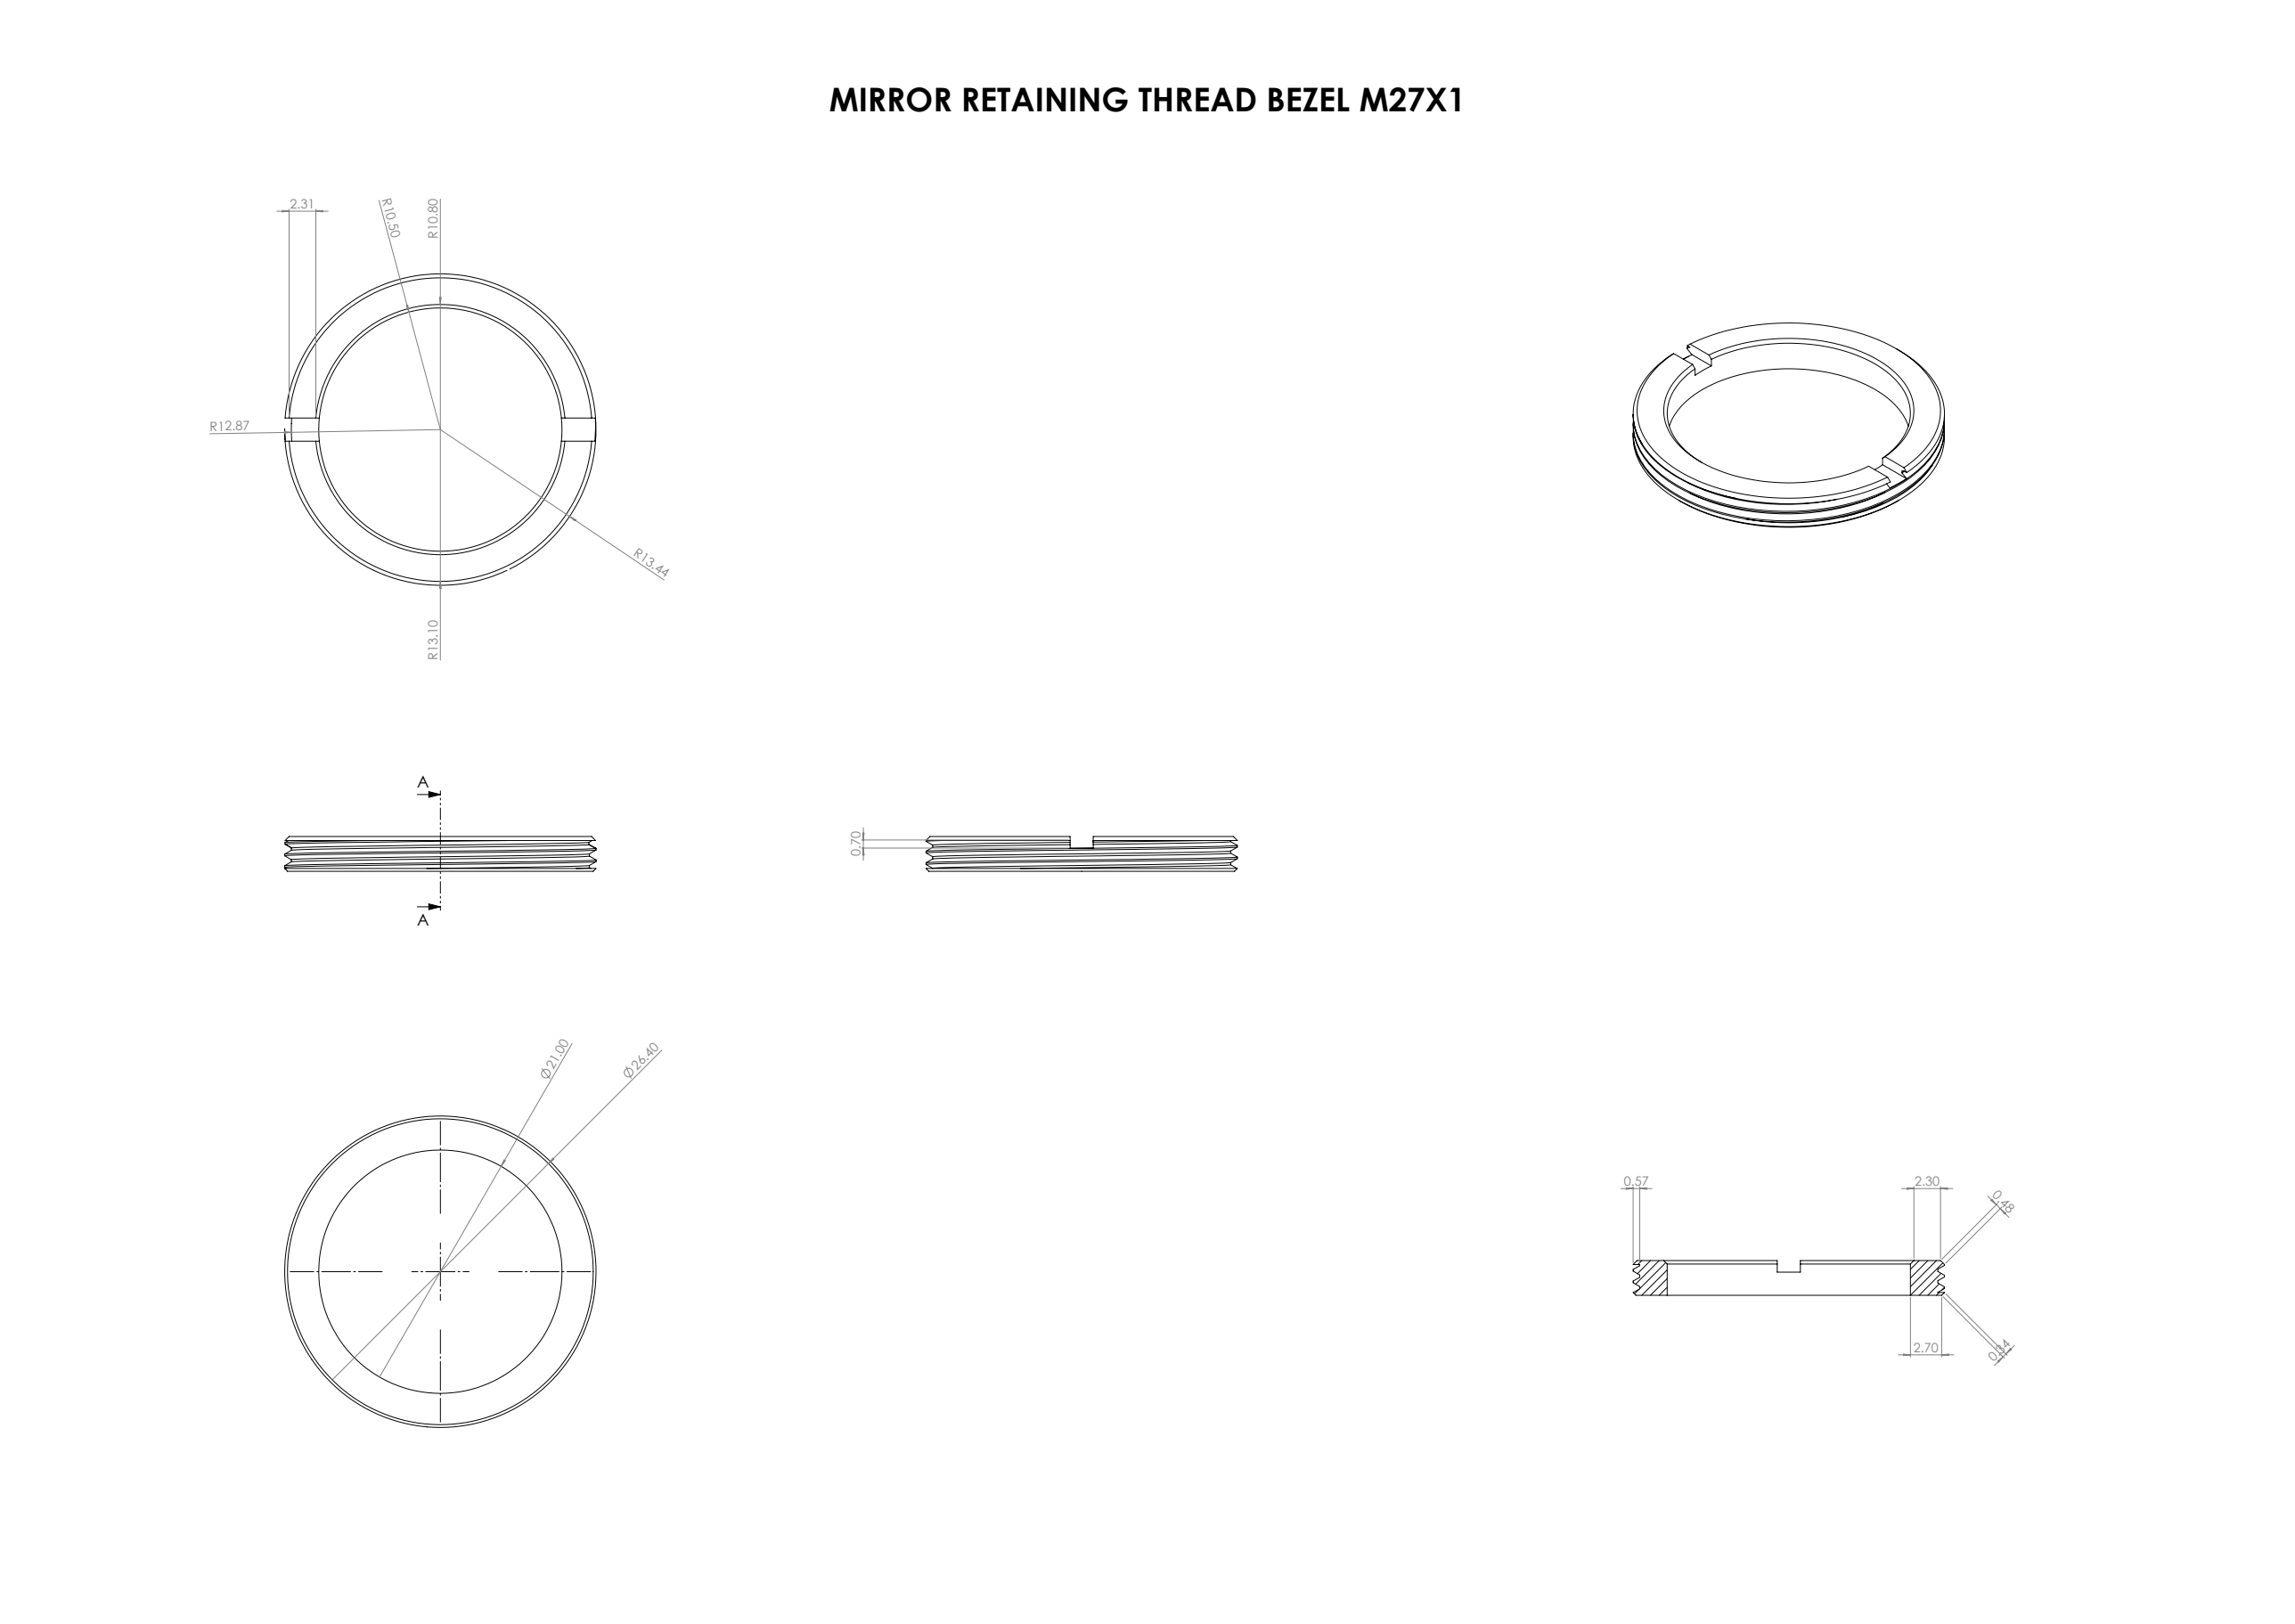
ISO-10303-21;
HEADER;
/* Generated by software containing ST-Developer
 * from STEP Tools, Inc. (www.steptools.com) 
 */

FILE_DESCRIPTION(
/* description */ (''),
/* implementation_level */ '2;1');

FILE_NAME(
/* name */ 
'07_Mirror_Retaining_Thread_Bezel_M27x1.step',
/* time_stamp */ '2026-10-20T10:06:23-07:00',
/* author */ (''),
/* organization */ (''),
/* preprocessor_version */ 'ST-DEVELOPER v20.2',
/* originating_system */ 'Autodesk Translation Framework v15.15.0.0',
/* authorisation */ '');

FILE_SCHEMA (('AUTOMOTIVE_DESIGN { 1 0 10303 214 3 1 1 }'));
ENDSEC;

DATA;
#10=MECHANICAL_DESIGN_GEOMETRIC_PRESENTATION_REPRESENTATION('',(#465),#38611);
#98=(
BOUNDED_CURVE()
B_SPLINE_CURVE(2,(#24495,#24496,#24497),.UNSPECIFIED.,.F.,.F.)
B_SPLINE_CURVE_WITH_KNOTS((3,3),(0.,0.048540461555457),.UNSPECIFIED.)
CURVE()
GEOMETRIC_REPRESENTATION_ITEM()
RATIONAL_B_SPLINE_CURVE((1.,1.0000974490119,1.00002789674321))
REPRESENTATION_ITEM('')
);
#99=(
BOUNDED_CURVE()
B_SPLINE_CURVE(2,(#24501,#24502,#24503),.UNSPECIFIED.,.F.,.F.)
B_SPLINE_CURVE_WITH_KNOTS((3,3),(0.,0.0425206671334367),.UNSPECIFIED.)
CURVE()
GEOMETRIC_REPRESENTATION_ITEM()
RATIONAL_B_SPLINE_CURVE((1.,1.00010008479633,1.))
REPRESENTATION_ITEM('')
);
#100=(
BOUNDED_CURVE()
B_SPLINE_CURVE(2,(#24513,#24514,#24515),.UNSPECIFIED.,.F.,.F.)
B_SPLINE_CURVE_WITH_KNOTS((3,3),(0.,0.0425206671334366),.UNSPECIFIED.)
CURVE()
GEOMETRIC_REPRESENTATION_ITEM()
RATIONAL_B_SPLINE_CURVE((1.,1.00010008445539,1.))
REPRESENTATION_ITEM('')
);
#101=(
BOUNDED_CURVE()
B_SPLINE_CURVE(2,(#24518,#24519,#24520),.UNSPECIFIED.,.F.,.F.)
B_SPLINE_CURVE_WITH_KNOTS((3,3),(0.00810844555795414,0.0566489071109945),
 .UNSPECIFIED.)
CURVE()
GEOMETRIC_REPRESENTATION_ITEM()
RATIONAL_B_SPLINE_CURVE((1.00002789660287,1.00009744852162,1.))
REPRESENTATION_ITEM('')
);
#102=(
BOUNDED_CURVE()
B_SPLINE_CURVE(2,(#24534,#24535,#24536),.UNSPECIFIED.,.F.,.F.)
B_SPLINE_CURVE_WITH_KNOTS((3,3),(0.,0.0485404615530411),.UNSPECIFIED.)
CURVE()
GEOMETRIC_REPRESENTATION_ITEM()
RATIONAL_B_SPLINE_CURVE((1.,1.00009744852162,1.00002789660287))
REPRESENTATION_ITEM('')
);
#103=(
BOUNDED_CURVE()
B_SPLINE_CURVE(2,(#24540,#24541,#24542),.UNSPECIFIED.,.F.,.F.)
B_SPLINE_CURVE_WITH_KNOTS((3,3),(0.,0.0425206671334366),.UNSPECIFIED.)
CURVE()
GEOMETRIC_REPRESENTATION_ITEM()
RATIONAL_B_SPLINE_CURVE((1.,1.00010008445539,1.))
REPRESENTATION_ITEM('')
);
#104=(
BOUNDED_CURVE()
B_SPLINE_CURVE(2,(#24552,#24553,#24554),.UNSPECIFIED.,.F.,.F.)
B_SPLINE_CURVE_WITH_KNOTS((3,3),(0.,0.0425206671334367),.UNSPECIFIED.)
CURVE()
GEOMETRIC_REPRESENTATION_ITEM()
RATIONAL_B_SPLINE_CURVE((1.,1.00010008479633,1.))
REPRESENTATION_ITEM('')
);
#105=(
BOUNDED_CURVE()
B_SPLINE_CURVE(2,(#24557,#24558,#24559),.UNSPECIFIED.,.F.,.F.)
B_SPLINE_CURVE_WITH_KNOTS((3,3),(0.00810844555553747,0.0566489071109946),
 .UNSPECIFIED.)
CURVE()
GEOMETRIC_REPRESENTATION_ITEM()
RATIONAL_B_SPLINE_CURVE((1.00002789674321,1.0000974490119,1.))
REPRESENTATION_ITEM('')
);
#437=SHAPE_REPRESENTATION_RELATIONSHIP('SRR','None',#38673,#451);
#451=ADVANCED_BREP_SHAPE_REPRESENTATION('',(#479),#38602);
#465=STYLED_ITEM('',(#38871),#479);
#479=MANIFOLD_SOLID_BREP('Ring',#16239);
#492=B_SPLINE_SURFACE_WITH_KNOTS('',3,3,((#23661,#23662,#23663,#23664,#23665,
#23666,#23667,#23668,#23669,#23670,#23671,#23672,#23673,#23674,#23675,#23676,
#23677,#23678,#23679,#23680,#23681,#23682,#23683,#23684,#23685,#23686,#23687,
#23688,#23689,#23690,#23691,#23692,#23693,#23694,#23695,#23696,#23697),
(#23698,#23699,#23700,#23701,#23702,#23703,#23704,#23705,#23706,#23707,
#23708,#23709,#23710,#23711,#23712,#23713,#23714,#23715,#23716,#23717,#23718,
#23719,#23720,#23721,#23722,#23723,#23724,#23725,#23726,#23727,#23728,#23729,
#23730,#23731,#23732,#23733,#23734),(#23735,#23736,#23737,#23738,#23739,
#23740,#23741,#23742,#23743,#23744,#23745,#23746,#23747,#23748,#23749,#23750,
#23751,#23752,#23753,#23754,#23755,#23756,#23757,#23758,#23759,#23760,#23761,
#23762,#23763,#23764,#23765,#23766,#23767,#23768,#23769,#23770,#23771),
(#23772,#23773,#23774,#23775,#23776,#23777,#23778,#23779,#23780,#23781,
#23782,#23783,#23784,#23785,#23786,#23787,#23788,#23789,#23790,#23791,#23792,
#23793,#23794,#23795,#23796,#23797,#23798,#23799,#23800,#23801,#23802,#23803,
#23804,#23805,#23806,#23807,#23808)),.UNSPECIFIED.,.F.,.F.,.F.,(4,4),(4,
1,1,1,1,1,1,1,1,1,1,1,1,1,1,1,1,1,1,1,1,1,1,1,1,1,1,1,1,1,1,1,1,1,4),(0.,
0.0661932083625904),(9.4992404446547,9.97150665008959,10.4437728555245,
10.9160390609594,11.3883052663942,11.8605714718291,12.332837677264,12.8051038826989,
13.2773700881338,13.7496362935687,14.2219024990035,14.6941687044384,15.1664349098733,
15.6387011153082,16.1109673207431,16.583233526178,17.0554997316128,17.5277659370477,
18.0000321424826,18.4722983479175,18.9445645533524,19.4168307587873,19.8890969642221,
20.361363169657,20.8336293750919,21.3058955805268,21.7781617859617,22.2504279913965,
22.7226941968314,23.1949604022663,23.6672266077012,24.1394928131361,24.611759018571,
25.0840252240059,25.5562914294407),.UNSPECIFIED.);
#493=B_SPLINE_SURFACE_WITH_KNOTS('',3,3,((#24122,#24123,#24124,#24125,#24126,
#24127,#24128,#24129,#24130,#24131,#24132,#24133,#24134,#24135,#24136,#24137,
#24138,#24139,#24140,#24141,#24142,#24143,#24144,#24145,#24146,#24147,#24148,
#24149,#24150,#24151,#24152),(#24153,#24154,#24155,#24156,#24157,#24158,
#24159,#24160,#24161,#24162,#24163,#24164,#24165,#24166,#24167,#24168,#24169,
#24170,#24171,#24172,#24173,#24174,#24175,#24176,#24177,#24178,#24179,#24180,
#24181,#24182,#24183),(#24184,#24185,#24186,#24187,#24188,#24189,#24190,
#24191,#24192,#24193,#24194,#24195,#24196,#24197,#24198,#24199,#24200,#24201,
#24202,#24203,#24204,#24205,#24206,#24207,#24208,#24209,#24210,#24211,#24212,
#24213,#24214),(#24215,#24216,#24217,#24218,#24219,#24220,#24221,#24222,
#24223,#24224,#24225,#24226,#24227,#24228,#24229,#24230,#24231,#24232,#24233,
#24234,#24235,#24236,#24237,#24238,#24239,#24240,#24241,#24242,#24243,#24244,
#24245)),.UNSPECIFIED.,.F.,.F.,.F.,(4,4),(4,1,1,1,1,1,1,1,1,1,1,1,1,1,1,
1,1,1,1,1,1,1,1,1,1,1,1,1,4),(0.,0.0661932083625904),(15.7493687799271,
16.2181316635384,16.6868945471497,17.155657430761,17.6244203143723,18.0931831979836,
18.5619460815949,19.0307089652062,19.4994718488175,19.9682347324288,20.4369976160401,
20.9057604996514,21.3745233832627,21.8432862668739,22.3120491504852,22.7808120340965,
23.2495749177078,23.7183378013191,24.1871006849304,24.6558635685417,25.124626452153,
25.5933893357643,26.0621522193756,26.5309151029869,26.9996779865982,27.4684408702095,
27.9372037538208,28.4059666374321,28.8747295210434),.UNSPECIFIED.);
#494=B_SPLINE_SURFACE_WITH_KNOTS('',3,3,((#24347,#24348,#24349,#24350,#24351,
#24352,#24353,#24354,#24355),(#24356,#24357,#24358,#24359,#24360,#24361,
#24362,#24363,#24364),(#24365,#24366,#24367,#24368,#24369,#24370,#24371,
#24372,#24373),(#24374,#24375,#24376,#24377,#24378,#24379,#24380,#24381,
#24382)),.UNSPECIFIED.,.F.,.F.,.F.,(4,4),(4,1,1,1,1,1,4),(0.,0.0661932083625904),
(12.6424782450754,12.9748140827407,13.6394857580714,13.9718215957368,14.6364932710675,
15.3011649463983,15.6335007840636),.UNSPECIFIED.);
#495=B_SPLINE_SURFACE_WITH_KNOTS('',3,3,((#24418,#24419,#24420,#24421,#24422),
(#24423,#24424,#24425,#24426,#24427),(#24428,#24429,#24430,#24431,#24432),
(#24433,#24434,#24435,#24436,#24437)),.UNSPECIFIED.,.F.,.F.,.F.,(4,4),(4,
1,4),(0.0383415492497091,0.0661932083625904),(11.6150328478183,11.9900267092154,
12.4900185244115),.UNSPECIFIED.);
#496=B_SPLINE_SURFACE_WITH_KNOTS('',3,3,((#24459,#24460,#24461,#24462,#24463),
(#24464,#24465,#24466,#24467,#24468),(#24469,#24470,#24471,#24472,#24473),
(#24474,#24475,#24476,#24477,#24478)),.UNSPECIFIED.,.F.,.F.,.F.,(4,4),(4,
1,4),(0.0327046027417864,0.0661932083625904),(8.2965947562157,8.82345511654988,
9.35031547688406),.UNSPECIFIED.);
#528=B_SPLINE_CURVE_WITH_KNOTS('',3,(#23411,#23412,#23413,#23414,#23415,
#23416,#23417,#23418,#23419,#23420,#23421,#23422,#23423,#23424,#23425,#23426,
#23427,#23428,#23429,#23430,#23431,#23432,#23433,#23434,#23435,#23436,#23437,
#23438,#23439,#23440,#23441,#23442,#23443,#23444,#23445,#23446,#23447,#23448,
#23449,#23450,#23451,#23452,#23453),.UNSPECIFIED.,.F.,.F.,(4,3,3,3,3,3,
3,3,3,3,3,3,3,3,4),(-10.3761157273102,-10.2282534190556,-9.75949053544433,
-9.29072765183303,-8.82196476822174,-8.35320188461044,-7.88443900099915,
-7.41567611738786,-6.94691323377656,-6.47815035016526,-6.00938746655397,
-5.54062458294268,-5.07186169933138,-4.60309881572009,-4.16739290401597),
 .UNSPECIFIED.);
#529=B_SPLINE_CURVE_WITH_KNOTS('',3,(#23456,#23457,#23458,#23459,#23460,
#23461,#23462,#23463,#23464,#23465,#23466,#23467,#23468,#23469,#23470,#23471,
#23472,#23473,#23474,#23475,#23476,#23477,#23478,#23479,#23480,#23481,#23482,
#23483,#23484,#23485,#23486,#23487,#23488,#23489,#23490,#23491,#23492,#23493,
#23494,#23495,#23496,#23497,#23498),.UNSPECIFIED.,.F.,.F.,(4,3,3,3,3,3,
3,3,3,3,3,3,3,3,4),(1.20264568843901,1.67491189387389,2.14717809930877,
2.61944430474366,3.09171051017854,3.56397671561342,4.03624292104831,4.50850912648319,
4.98077533191807,5.45304153735295,5.92530774278784,6.39757394822272,6.8698401536576,
7.34210635909249,7.41136851173327),.UNSPECIFIED.);
#530=B_SPLINE_CURVE_WITH_KNOTS('',3,(#23503,#23504,#23505,#23506,#23507,
#23508,#23509,#23510,#23511,#23512,#23513,#23514,#23515,#23516,#23517,#23518,
#23519,#23520,#23521,#23522,#23523,#23524,#23525,#23526,#23527,#23528,#23529,
#23530,#23531,#23532,#23533,#23534,#23535,#23536,#23537,#23538,#23539,#23540,
#23541,#23542,#23543,#23544,#23545),.UNSPECIFIED.,.F.,.F.,(4,3,3,3,3,3,
3,3,3,3,3,3,3,3,4),(-16.6593010344898,-16.3221709060024,-15.8534080223912,
-15.3846451387799,-14.9158822551686,-14.4471193715573,-13.978356487946,
-13.5095936043347,-13.0408307207234,-12.5720678371121,-12.1033049535008,
-11.6345420698895,-11.1657791862782,-10.6970163026669,-10.3761157273102),
 .UNSPECIFIED.);
#531=B_SPLINE_CURVE_WITH_KNOTS('',3,(#23546,#23547,#23548,#23549,#23550,
#23551,#23552,#23553,#23554,#23555,#23556,#23557,#23558,#23559,#23560,#23561,
#23562,#23563,#23564,#23565,#23566,#23567,#23568,#23569,#23570,#23571,#23572,
#23573,#23574,#23575,#23576,#23577,#23578,#23579,#23580,#23581,#23582,#23583,
#23584,#23585,#23586,#23587,#23588),.UNSPECIFIED.,.F.,.F.,(4,3,3,3,3,3,
3,3,3,3,3,3,3,3,4),(7.41136851173327,7.81437256452737,8.28663876996226,
8.75890497539714,9.23117118083202,9.7034373862669,10.1757035917018,10.6479697971367,
11.1202360025716,11.5925022080064,12.0647684134413,12.5370346188762,13.0093008243111,
13.481567029746,13.6945538189129),.UNSPECIFIED.);
#532=B_SPLINE_CURVE_WITH_KNOTS('',3,(#23594,#23595,#23596,#23597,#23598,
#23599,#23600,#23601,#23602,#23603,#23604,#23605,#23606,#23607),
 .UNSPECIFIED.,.F.,.F.,(4,1,1,1,1,1,1,1,1,1,1,4),(21.9911485751285,22.3120491504852,
22.7808120340965,23.2495749177078,23.7183378013191,24.1871006849304,24.6558635685417,
25.124626452153,25.5933893357643,26.0621522193756,26.5309151029869,26.7952085499488),
 .UNSPECIFIED.);
#533=B_SPLINE_CURVE_WITH_KNOTS('',3,(#23610,#23611,#23612,#23613,#23614,
#23615,#23616,#23617,#23618,#23619,#23620),.UNSPECIFIED.,.F.,.F.,(4,1,1,
1,1,1,1,1,4),(21.9911485751285,22.2504279913965,22.7226941968314,23.1949604022663,
23.6672266077012,24.1394928131361,24.611759018571,25.0840252240059,25.5562914294407),
 .UNSPECIFIED.);
#534=B_SPLINE_CURVE_WITH_KNOTS('',3,(#23627,#23628,#23629,#23630,#23631,
#23632,#23633,#23634,#23635,#23636,#23637,#23638,#23639,#23640,#23641,#23642,
#23643),.UNSPECIFIED.,.F.,.F.,(4,1,1,1,1,1,1,1,1,1,1,1,1,1,4),(15.7493687799271,
16.2181316635384,16.6868945471497,17.155657430761,17.6244203143723,18.0931831979836,
18.5619460815949,19.0307089652062,19.4994718488175,19.9682347324288,20.4369976160401,
20.9057604996514,21.3745233832627,21.8432862668739,21.9911485751285),
 .UNSPECIFIED.);
#535=B_SPLINE_CURVE_WITH_KNOTS('',3,(#23644,#23645,#23646,#23647,#23648,
#23649,#23650,#23651,#23652,#23653,#23654,#23655,#23656,#23657,#23658,#23659,
#23660),.UNSPECIFIED.,.F.,.F.,(4,1,1,1,1,1,1,1,1,1,1,1,1,1,4),(15.707963267949,
16.1109673207431,16.583233526178,17.0554997316128,17.5277659370477,18.0000321424826,
18.4722983479175,18.9445645533524,19.4168307587873,19.8890969642221,20.361363169657,
20.8336293750919,21.3058955805268,21.7781617859617,21.9911485751285),
 .UNSPECIFIED.);
#536=B_SPLINE_CURVE_WITH_KNOTS('',3,(#23811,#23812,#23813,#23814,#23815,
#23816),.UNSPECIFIED.,.F.,.F.,(4,2,4),(0.00194275133685398,0.0331760695218423,
0.0663555691945392),.UNSPECIFIED.);
#537=B_SPLINE_CURVE_WITH_KNOTS('',3,(#23818,#23819,#23820,#23821,#23822,
#23823,#23824),.UNSPECIFIED.,.F.,.F.,(4,3,4),(0.0503544158881505,0.216395299739162,
0.250849009142881),.UNSPECIFIED.);
#538=B_SPLINE_CURVE_WITH_KNOTS('',3,(#23826,#23827,#23828,#23829,#23830,
#23831),.UNSPECIFIED.,.F.,.F.,(4,2,4),(0.,0.0331528039224116,0.0596005631617877),
 .UNSPECIFIED.);
#539=B_SPLINE_CURVE_WITH_KNOTS('',3,(#23832,#23833,#23834,#23835,#23836,
#23837,#23838,#23839,#23840,#23841,#23842),.UNSPECIFIED.,.F.,.F.,(4,1,1,
1,1,1,1,1,4),(12.644156658622,12.8051038826989,13.2773700881338,13.7496362935687,
14.2219024990035,14.6941687044384,15.1664349098733,15.6387011153082,15.707963267949),
 .UNSPECIFIED.);
#540=B_SPLINE_CURVE_WITH_KNOTS('',3,(#23844,#23845,#23846,#23847,#23848,
#23849,#23850,#23851,#23852,#23853,#23854,#23855,#23856,#23857,#23858,#23859,
#23860,#23861,#23862,#23863,#23864,#23865,#23866,#23867,#23868,#23869,#23870,
#23871,#23872,#23873,#23874,#23875,#23876,#23877,#23878,#23879,#23880,#23881,
#23882,#23883,#23884,#23885,#23886,#23887,#23888,#23889,#23890,#23891,#23892,
#23893,#23894,#23895,#23896,#23897,#23898,#23899,#23900,#23901,#23902,#23903,
#23904,#23905,#23906,#23907,#23908,#23909,#23910,#23911,#23912,#23913,#23914,
#23915,#23916,#23917,#23918,#23919,#23920,#23921,#23922,#23923,#23924,#23925),
 .UNSPECIFIED.,.F.,.F.,(4,3,3,3,3,3,3,3,3,3,3,3,3,3,3,3,3,3,3,3,3,3,3,3,
3,3,3,4),(-2.74250302776518,-2.57686990184093,-2.48672838486568,-2.42438465251614,
-2.38771591000872,-2.22247456456748,-2.11726591049527,-2.05259329034323,
-2.02076827609199,-1.85670314451872,-1.69196748309613,-1.57688547236148,
-1.53552332264269,-1.50624221680821,-1.3425714308067,-1.23163944015751,
-1.07689892021046,-1.03296271663657,-0.9930706972102,-0.830572896985994,
-0.668873173603195,-0.612677360369303,-0.533465071065458,-0.502301898288595,
-0.34107686385133,-0.179301278866167,-0.0205350393876634,0.),
 .UNSPECIFIED.);
#541=B_SPLINE_CURVE_WITH_KNOTS('',3,(#23926,#23927,#23928,#23929,#23930,
#23931,#23932,#23933,#23934,#23935,#23936,#23937,#23938),.UNSPECIFIED.,
 .F.,.F.,(4,3,3,3,4),(13.6945538189129,13.9538332351809,14.4260994406157,
14.8983656460506,15.1801757021305),.UNSPECIFIED.);
#542=B_SPLINE_CURVE_WITH_KNOTS('',3,(#23940,#23941,#23942,#23943,#23944,
#23945),.UNSPECIFIED.,.F.,.F.,(4,2,4),(0.0278987519445973,0.0331528039168248,
0.0663033314332046),.UNSPECIFIED.);
#543=B_SPLINE_CURVE_WITH_KNOTS('',3,(#23947,#23948,#23949,#23950,#23951,
#23952,#23953,#23954,#23955,#23956,#23957,#23958,#23959,#23960,#23961,#23962,
#23963,#23964,#23965,#23966,#23967,#23968,#23969,#23970,#23971,#23972,#23973,
#23974,#23975,#23976,#23977,#23978,#23979,#23980),.UNSPECIFIED.,.F.,.F.,
(4,3,3,3,3,3,3,3,3,3,3,4),(-2.7450049110565,-2.58394001349979,-2.45527459604387,
-2.40771262127862,-2.37283567347439,-2.22079245860333,-2.1259413782344,
-2.07191392018567,-2.04033511913998,-1.8778682623923,-1.71515635324971,
-1.60487049281501),.UNSPECIFIED.);
#544=B_SPLINE_CURVE_WITH_KNOTS('',3,(#23981,#23982,#23983,#23984,#23985,
#23986,#23987,#23988,#23989),.UNSPECIFIED.,.F.,.F.,(4,1,1,1,1,1,4),(10.3761157273102,
10.4437728555245,10.9160390609594,11.3883052663942,11.8605714718291,12.332837677264,
12.4885845700963),.UNSPECIFIED.);
#545=B_SPLINE_CURVE_WITH_KNOTS('',3,(#23996,#23997,#23998,#23999,#24000,
#24001,#24002,#24003,#24004,#24005,#24006,#24007,#24008,#24009,#24010,#24011,
#24012,#24013,#24014,#24015,#24016,#24017,#24018,#24019,#24020,#24021,#24022,
#24023,#24024,#24025,#24026,#24027,#24028,#24029,#24030,#24031,#24032,#24033,
#24034,#24035,#24036,#24037,#24038),.UNSPECIFIED.,.F.,.F.,(4,3,3,3,3,3,
3,3,3,3,3,3,3,3,4),(-2.74250302776508,-2.66850832126571,-2.50265052845,
-2.39214152203743,-2.35757539427899,-2.19175335172764,-2.08902158205883,
-2.04611352983189,-2.01171973266703,-1.84702980906273,-1.78082627305242,
-1.61618310024309,-1.53556392179723,-1.50606805204129,-1.3410808692064),
 .UNSPECIFIED.);
#546=B_SPLINE_CURVE_WITH_KNOTS('',3,(#24047,#24048,#24049,#24050,#24051,
#24052,#24053,#24054,#24055,#24056,#24057,#24058,#24059,#24060,#24061,#24062,
#24063,#24064,#24065,#24066,#24067,#24068,#24069,#24070,#24071,#24072,#24073,
#24074,#24075,#24076,#24077,#24078,#24079,#24080),.UNSPECIFIED.,.F.,.F.,
(4,3,3,3,3,3,3,3,3,3,3,4),(-1.14003686198146,-1.05830319525406,-1.0207818545891,
-0.992096849082759,-0.829622775007598,-0.666879442976059,-0.576523485569153,
-0.520860847165652,-0.486167528162247,-0.325408793834023,-0.162704396917011,
0.),.UNSPECIFIED.);
#547=B_SPLINE_CURVE_WITH_KNOTS('',3,(#24087,#24088,#24089,#24090,#24091,
#24092,#24093,#24094,#24095,#24096,#24097,#24098,#24099,#24100,#24101,#24102,
#24103,#24104,#24105,#24106,#24107,#24108,#24109,#24110,#24111,#24112,#24113,
#24114,#24115,#24116,#24117,#24118,#24119,#24120),.UNSPECIFIED.,.F.,.F.,
(4,3,3,3,3,3,3,3,3,3,3,4),(-1.40414311178045,-1.24106650608481,-1.10748442566693,
-1.06335789746563,-1.02152275246228,-0.856189859529963,-0.706738184413317,
-0.541595540057656,-0.502301503557962,-0.336744830409687,-0.168372415204844,
0.),.UNSPECIFIED.);
#548=B_SPLINE_CURVE_WITH_KNOTS('',3,(#24247,#24248,#24249,#24250,#24251,
#24252),.UNSPECIFIED.,.F.,.F.,(4,2,4),(0.,0.0331760695065475,0.0651963829308363),
 .UNSPECIFIED.);
#549=B_SPLINE_CURVE_WITH_KNOTS('',3,(#24254,#24255,#24256,#24257,#24258,
#24259,#24260),.UNSPECIFIED.,.F.,.F.,(4,3,4),(-17.259696673225,-16.7909337896137,
-16.6593010344898),.UNSPECIFIED.);
#550=B_SPLINE_CURVE_WITH_KNOTS('',3,(#24261,#24262,#24263,#24264,#24265,
#24266,#24267,#24268,#24269,#24270,#24271,#24272,#24273,#24274,#24275,#24276,
#24277,#24278,#24279,#24280,#24281,#24282,#24283,#24284,#24285,#24286,#24287,
#24288,#24289,#24290,#24291,#24292,#24293,#24294,#24295,#24296,#24297,#24298,
#24299,#24300,#24301,#24302,#24303,#24304,#24305,#24306,#24307,#24308,#24309,
#24310,#24311,#24312,#24313,#24314,#24315,#24316,#24317,#24318,#24319,#24320,
#24321,#24322,#24323,#24324,#24325,#24326,#24327,#24328,#24329,#24330,#24331,
#24332,#24333,#24334,#24335,#24336,#24337,#24338,#24339,#24340,#24341,#24342),
 .UNSPECIFIED.,.F.,.F.,(4,3,3,3,3,3,3,3,3,3,3,3,3,3,3,3,3,3,3,3,3,3,3,3,
3,3,3,4),(-2.74500491105659,-2.58350402394403,-2.48061289382144,-2.41107509153194,
-2.37265853925204,-2.21067382092066,-2.12552001520103,-2.08101176042865,
-2.04586716316976,-1.88271537722459,-1.87005859804212,-1.7095303618963,
-1.59527874414824,-1.55981736007669,-1.52718746411221,-1.36294474918432,
-1.25252389090405,-1.09667110605016,-1.05462433202708,-1.02403188127795,
-0.859632450592286,-0.694838694901999,-0.629112751488469,-0.545267156057735,
-0.502057707499426,-0.336851513025011,-0.168425756512506,0.),
 .UNSPECIFIED.);
#551=B_SPLINE_CURVE_WITH_KNOTS('',3,(#24343,#24344,#24345,#24346),
 .UNSPECIFIED.,.F.,.F.,(4,4),(0.0501531527093442,0.0969267489892359),
 .UNSPECIFIED.);
#552=B_SPLINE_CURVE_WITH_KNOTS('',3,(#24384,#24385,#24386,#24387),
 .UNSPECIFIED.,.F.,.F.,(4,4),(0.0335690789016969,0.0663555691090524),
 .UNSPECIFIED.);
#553=B_SPLINE_CURVE_WITH_KNOTS('',3,(#24389,#24390,#24391,#24392,#24393,
#24394,#24395,#24396,#24397,#24398,#24399,#24400,#24401),.UNSPECIFIED.,
 .F.,.F.,(4,3,3,3,4),(-4.01846793624531,-3.68613209857994,-3.02146042324921,
-2.35678874791848,-2.07952097109452),.UNSPECIFIED.);
#554=B_SPLINE_CURVE_WITH_KNOTS('',3,(#24403,#24404,#24405,#24406,#24407,
#24408),.UNSPECIFIED.,.F.,.F.,(4,2,4),(0.,0.0331528039173847,0.0663033314433819),
 .UNSPECIFIED.);
#555=B_SPLINE_CURVE_WITH_KNOTS('',3,(#24409,#24410,#24411,#24412,#24413,
#24414,#24415,#24416,#24417),.UNSPECIFIED.,.F.,.F.,(4,1,1,1,1,1,4),(12.644156658622,
12.9748140827407,13.6394857580714,13.9718215957368,14.6364932710675,15.3011649463983,
15.6301772236861),.UNSPECIFIED.);
#556=B_SPLINE_CURVE_WITH_KNOTS('',3,(#24439,#24440,#24441,#24442),
 .UNSPECIFIED.,.F.,.F.,(4,4),(0.,0.0278987520022068),.UNSPECIFIED.);
#557=B_SPLINE_CURVE_WITH_KNOTS('',3,(#24443,#24444,#24445,#24446,#24447),
 .UNSPECIFIED.,.F.,.F.,(4,1,4),(11.6150328478183,11.9900267092154,12.4885845700963),
 .UNSPECIFIED.);
#558=B_SPLINE_CURVE_WITH_KNOTS('',3,(#24480,#24481,#24482,#24483,#24484,
#24485),.UNSPECIFIED.,.F.,.F.,(4,2,4),(0.,0.0331760694937226,0.0335690788757423),
 .UNSPECIFIED.);
#559=B_SPLINE_CURVE_WITH_KNOTS('',3,(#24486,#24487,#24488,#24489,#24490,
#24491,#24492),.UNSPECIFIED.,.F.,.F.,(4,3,4),(0.,0.52686036033418,1.05372072066836),
 .UNSPECIFIED.);
#907=CYLINDRICAL_SURFACE('',#16785,1.3442);
#908=CYLINDRICAL_SURFACE('',#16786,1.3442);
#909=CYLINDRICAL_SURFACE('',#16787,1.286875);
#910=CYLINDRICAL_SURFACE('',#16789,1.286875);
#911=CYLINDRICAL_SURFACE('',#16798,1.286875);
#912=CYLINDRICAL_SURFACE('',#16800,1.286875);
#913=CYLINDRICAL_SURFACE('',#16806,1.3442);
#914=CYLINDRICAL_SURFACE('',#16808,1.3442);
#915=CYLINDRICAL_SURFACE('',#16817,1.05);
#1185=FACE_BOUND('',#2990,.T.);
#1341=CIRCLE('',#16788,1.286875);
#1342=CIRCLE('',#16790,1.286875);
#1343=CIRCLE('',#16792,1.3442);
#1344=CIRCLE('',#16794,1.3442);
#1345=CIRCLE('',#16795,1.286875);
#1346=CIRCLE('',#16797,1.3442);
#1347=CIRCLE('',#16799,1.286875);
#1348=CIRCLE('',#16802,1.3442);
#1349=CIRCLE('',#16803,1.3442);
#1350=CIRCLE('',#16807,1.3442);
#1351=CIRCLE('',#16809,1.3442);
#1352=CIRCLE('',#16811,1.05);
#1353=CIRCLE('',#16812,1.05);
#1354=CIRCLE('',#16815,1.05);
#1355=CIRCLE('',#16818,1.05);
#1356=CIRCLE('',#16819,1.05);
#1357=CIRCLE('',#16820,1.05);
#1358=CIRCLE('',#16822,1.31);
#1359=CIRCLE('',#16824,1.31);
#1360=CIRCLE('',#16826,1.08);
#1361=CIRCLE('',#16828,1.08);
#1362=CIRCLE('',#16832,1.32);
#1735=CONICAL_SURFACE('',#16821,1.33,0.785398163397449);
#1736=CONICAL_SURFACE('',#16823,1.33,0.785398163397449);
#1737=CONICAL_SURFACE('',#16829,1.065,0.785398163397447);
#1738=CONICAL_SURFACE('',#16830,1.065,0.785398163397447);
#1739=CONICAL_SURFACE('',#16831,1.335,0.785398163397448);
#2015=FACE_OUTER_BOUND('',#2958,.T.);
#2016=FACE_OUTER_BOUND('',#2959,.T.);
#2017=FACE_OUTER_BOUND('',#2960,.T.);
#2018=FACE_OUTER_BOUND('',#2961,.T.);
#2019=FACE_OUTER_BOUND('',#2962,.T.);
#2020=FACE_OUTER_BOUND('',#2963,.T.);
#2021=FACE_OUTER_BOUND('',#2964,.T.);
#2022=FACE_OUTER_BOUND('',#2965,.T.);
#2023=FACE_OUTER_BOUND('',#2966,.T.);
#2024=FACE_OUTER_BOUND('',#2967,.T.);
#2025=FACE_OUTER_BOUND('',#2968,.T.);
#2026=FACE_OUTER_BOUND('',#2969,.T.);
#2027=FACE_OUTER_BOUND('',#2970,.T.);
#2028=FACE_OUTER_BOUND('',#2971,.T.);
#2029=FACE_OUTER_BOUND('',#2972,.T.);
#2030=FACE_OUTER_BOUND('',#2973,.T.);
#2031=FACE_OUTER_BOUND('',#2974,.T.);
#2032=FACE_OUTER_BOUND('',#2975,.T.);
#2033=FACE_OUTER_BOUND('',#2976,.T.);
#2034=FACE_OUTER_BOUND('',#2977,.T.);
#2035=FACE_OUTER_BOUND('',#2978,.T.);
#2036=FACE_OUTER_BOUND('',#2979,.T.);
#2037=FACE_OUTER_BOUND('',#2980,.T.);
#2038=FACE_OUTER_BOUND('',#2981,.T.);
#2039=FACE_OUTER_BOUND('',#2982,.T.);
#2040=FACE_OUTER_BOUND('',#2983,.T.);
#2041=FACE_OUTER_BOUND('',#2984,.T.);
#2042=FACE_OUTER_BOUND('',#2985,.T.);
#2043=FACE_OUTER_BOUND('',#2986,.T.);
#2044=FACE_OUTER_BOUND('',#2987,.T.);
#2045=FACE_OUTER_BOUND('',#2988,.T.);
#2046=FACE_OUTER_BOUND('',#2989,.T.);
#2958=EDGE_LOOP('',(#11187,#11188,#11189,#11190));
#2959=EDGE_LOOP('',(#11191,#11192,#11193,#11194));
#2960=EDGE_LOOP('',(#11195,#11196,#11197,#11198));
#2961=EDGE_LOOP('',(#11199,#11200,#11201,#11202,#11203));
#2962=EDGE_LOOP('',(#11204,#11205,#11206,#11207,#11208,#11209,#11210,#11211,
#11212,#11213,#11214,#11215,#11216));
#2963=EDGE_LOOP('',(#11217,#11218,#11219));
#2964=EDGE_LOOP('',(#11220,#11221,#11222,#11223,#11224,#11225));
#2965=EDGE_LOOP('',(#11226,#11227,#11228));
#2966=EDGE_LOOP('',(#11229,#11230,#11231,#11232,#11233,#11234,#11235,#11236));
#2967=EDGE_LOOP('',(#11237,#11238,#11239,#11240,#11241));
#2968=EDGE_LOOP('',(#11242,#11243,#11244));
#2969=EDGE_LOOP('',(#11245,#11246,#11247,#11248,#11249,#11250));
#2970=EDGE_LOOP('',(#11251,#11252,#11253,#11254));
#2971=EDGE_LOOP('',(#11255,#11256,#11257,#11258,#11259));
#2972=EDGE_LOOP('',(#11260,#11261,#11262));
#2973=EDGE_LOOP('',(#11263,#11264,#11265,#11266,#11267,#11268,#11269,#11270,
#11271));
#2974=EDGE_LOOP('',(#11272,#11273,#11274,#11275,#11276,#11277,#11278,#11279,
#11280));
#2975=EDGE_LOOP('',(#11281,#11282,#11283,#11284));
#2976=EDGE_LOOP('',(#11285,#11286,#11287,#11288));
#2977=EDGE_LOOP('',(#11289,#11290,#11291,#11292,#11293,#11294,#11295));
#2978=EDGE_LOOP('',(#11296,#11297,#11298,#11299,#11300,#11301,#11302,#11303,
#11304,#11305));
#2979=EDGE_LOOP('',(#11306,#11307,#11308,#11309));
#2980=EDGE_LOOP('',(#11310,#11311,#11312,#11313,#11314,#11315,#11316,#11317,
#11318));
#2981=EDGE_LOOP('',(#11319,#11320,#11321,#11322,#11323,#11324,#11325,#11326,
#11327,#11328,#11329,#11330));
#2982=EDGE_LOOP('',(#11331,#11332,#11333,#11334,#11335,#11336));
#2983=EDGE_LOOP('',(#11337,#11338,#11339,#11340));
#2984=EDGE_LOOP('',(#11341,#11342,#11343,#11344));
#2985=EDGE_LOOP('',(#11345,#11346,#11347,#11348));
#2986=EDGE_LOOP('',(#11349,#11350,#11351,#11352));
#2987=EDGE_LOOP('',(#11353,#11354,#11355,#11356));
#2988=EDGE_LOOP('',(#11357,#11358,#11359,#11360,#11361,#11362));
#2989=EDGE_LOOP('',(#11363));
#2990=EDGE_LOOP('',(#11364));
#4084=LINE('',#23409,#5308);
#4085=LINE('',#23455,#5309);
#4086=LINE('',#23502,#5310);
#4087=LINE('',#23592,#5311);
#4088=LINE('',#23624,#5312);
#4089=LINE('',#23993,#5313);
#4090=LINE('',#24041,#5314);
#4091=LINE('',#24045,#5315);
#4092=LINE('',#24085,#5316);
#4093=LINE('',#24449,#5317);
#4094=LINE('',#24451,#5318);
#4095=LINE('',#24454,#5319);
#4096=LINE('',#24499,#5320);
#4097=LINE('',#24505,#5321);
#4098=LINE('',#24506,#5322);
#4099=LINE('',#24509,#5323);
#4100=LINE('',#24511,#5324);
#4101=LINE('',#24517,#5325);
#4102=LINE('',#24524,#5326);
#4103=LINE('',#24528,#5327);
#4104=LINE('',#24538,#5328);
#4105=LINE('',#24543,#5329);
#4106=LINE('',#24547,#5330);
#4107=LINE('',#24550,#5331);
#4108=LINE('',#24556,#5332);
#4109=LINE('',#24563,#5333);
#4110=LINE('',#24579,#5334);
#5308=VECTOR('',#19001,1.35);
#5309=VECTOR('',#19002,1.);
#5310=VECTOR('',#19005,1.35);
#5311=VECTOR('',#19008,1.286875);
#5312=VECTOR('',#19013,1.286875);
#5313=VECTOR('',#19018,1.);
#5314=VECTOR('',#19023,1.);
#5315=VECTOR('',#19026,1.);
#5316=VECTOR('',#19031,1.);
#5317=VECTOR('',#19036,1.);
#5318=VECTOR('',#19037,1.);
#5319=VECTOR('',#19042,1.);
#5320=VECTOR('',#19051,1.);
#5321=VECTOR('',#19052,1.);
#5322=VECTOR('',#19053,1.);
#5323=VECTOR('',#19056,1.);
#5324=VECTOR('',#19057,1.);
#5325=VECTOR('',#19058,1.);
#5326=VECTOR('',#19065,1.);
#5327=VECTOR('',#19070,1.);
#5328=VECTOR('',#19077,1.);
#5329=VECTOR('',#19078,1.);
#5330=VECTOR('',#19083,1.);
#5331=VECTOR('',#19086,1.);
#5332=VECTOR('',#19087,1.);
#5333=VECTOR('',#19092,1.05);
#5334=VECTOR('',#19121,1.335);
#6463=VERTEX_POINT('',#23407);
#6464=VERTEX_POINT('',#23408);
#6465=VERTEX_POINT('',#23410);
#6466=VERTEX_POINT('',#23454);
#6467=VERTEX_POINT('',#23500);
#6468=VERTEX_POINT('',#23501);
#6469=VERTEX_POINT('',#23590);
#6470=VERTEX_POINT('',#23591);
#6471=VERTEX_POINT('',#23593);
#6472=VERTEX_POINT('',#23608);
#6473=VERTEX_POINT('',#23622);
#6474=VERTEX_POINT('',#23623);
#6475=VERTEX_POINT('',#23625);
#6476=VERTEX_POINT('',#23809);
#6477=VERTEX_POINT('',#23810);
#6478=VERTEX_POINT('',#23817);
#6479=VERTEX_POINT('',#23825);
#6480=VERTEX_POINT('',#23843);
#6481=VERTEX_POINT('',#23939);
#6482=VERTEX_POINT('',#23946);
#6483=VERTEX_POINT('',#23991);
#6484=VERTEX_POINT('',#23992);
#6485=VERTEX_POINT('',#23994);
#6486=VERTEX_POINT('',#24040);
#6487=VERTEX_POINT('',#24042);
#6488=VERTEX_POINT('',#24044);
#6489=VERTEX_POINT('',#24046);
#6490=VERTEX_POINT('',#24083);
#6491=VERTEX_POINT('',#24084);
#6492=VERTEX_POINT('',#24086);
#6493=VERTEX_POINT('',#24246);
#6494=VERTEX_POINT('',#24253);
#6495=VERTEX_POINT('',#24383);
#6496=VERTEX_POINT('',#24388);
#6497=VERTEX_POINT('',#24402);
#6498=VERTEX_POINT('',#24438);
#6499=VERTEX_POINT('',#24450);
#6500=VERTEX_POINT('',#24456);
#6501=VERTEX_POINT('',#24479);
#6502=VERTEX_POINT('',#24494);
#6503=VERTEX_POINT('',#24498);
#6504=VERTEX_POINT('',#24500);
#6505=VERTEX_POINT('',#24504);
#6506=VERTEX_POINT('',#24508);
#6507=VERTEX_POINT('',#24510);
#6508=VERTEX_POINT('',#24512);
#6509=VERTEX_POINT('',#24516);
#6510=VERTEX_POINT('',#24527);
#6511=VERTEX_POINT('',#24529);
#6512=VERTEX_POINT('',#24533);
#6513=VERTEX_POINT('',#24537);
#6514=VERTEX_POINT('',#24539);
#6515=VERTEX_POINT('',#24545);
#6516=VERTEX_POINT('',#24549);
#6517=VERTEX_POINT('',#24551);
#6518=VERTEX_POINT('',#24555);
#6519=VERTEX_POINT('',#24561);
#6520=VERTEX_POINT('',#24577);
#8209=EDGE_CURVE('',#6463,#6464,#4084,.T.);
#8210=EDGE_CURVE('',#6463,#6465,#528,.T.);
#8211=EDGE_CURVE('',#6465,#6466,#4085,.F.);
#8212=EDGE_CURVE('',#6466,#6464,#529,.T.);
#8213=EDGE_CURVE('',#6467,#6468,#4086,.T.);
#8214=EDGE_CURVE('',#6467,#6463,#530,.T.);
#8215=EDGE_CURVE('',#6464,#6468,#531,.T.);
#8216=EDGE_CURVE('',#6469,#6470,#4087,.T.);
#8217=EDGE_CURVE('',#6469,#6471,#532,.T.);
#8218=EDGE_CURVE('',#6472,#6471,#1341,.T.);
#8219=EDGE_CURVE('',#6470,#6472,#533,.T.);
#8220=EDGE_CURVE('',#6473,#6474,#4088,.T.);
#8221=EDGE_CURVE('',#6475,#6473,#1342,.T.);
#8222=EDGE_CURVE('',#6475,#6469,#534,.T.);
#8223=EDGE_CURVE('',#6474,#6470,#535,.T.);
#8224=EDGE_CURVE('',#6476,#6477,#536,.T.);
#8225=EDGE_CURVE('',#6478,#6476,#537,.T.);
#8226=EDGE_CURVE('',#6479,#6478,#538,.T.);
#8227=EDGE_CURVE('',#6479,#6474,#539,.T.);
#8228=EDGE_CURVE('',#6480,#6472,#540,.T.);
#8229=EDGE_CURVE('',#6468,#6480,#541,.T.);
#8230=EDGE_CURVE('',#6481,#6466,#542,.T.);
#8231=EDGE_CURVE('',#6482,#6481,#543,.T.);
#8232=EDGE_CURVE('',#6482,#6477,#544,.T.);
#8233=EDGE_CURVE('',#6483,#6484,#4089,.T.);
#8234=EDGE_CURVE('',#6483,#6485,#1343,.T.);
#8235=EDGE_CURVE('',#6485,#6484,#545,.T.);
#8236=EDGE_CURVE('',#6486,#6481,#4090,.T.);
#8237=EDGE_CURVE('',#6486,#6487,#1344,.T.);
#8238=EDGE_CURVE('',#6488,#6487,#4091,.T.);
#8239=EDGE_CURVE('',#6488,#6489,#546,.T.);
#8240=EDGE_CURVE('',#6489,#6482,#1345,.T.);
#8241=EDGE_CURVE('',#6490,#6491,#4092,.T.);
#8242=EDGE_CURVE('',#6490,#6492,#547,.T.);
#8243=EDGE_CURVE('',#6492,#6491,#1346,.T.);
#8244=EDGE_CURVE('',#6465,#6493,#548,.T.);
#8245=EDGE_CURVE('',#6494,#6467,#549,.T.);
#8246=EDGE_CURVE('',#6471,#6494,#550,.T.);
#8247=EDGE_CURVE('',#6493,#6475,#551,.T.);
#8248=EDGE_CURVE('',#6484,#6495,#552,.T.);
#8249=EDGE_CURVE('',#6496,#6485,#553,.T.);
#8250=EDGE_CURVE('',#6497,#6496,#554,.T.);
#8251=EDGE_CURVE('',#6495,#6497,#555,.T.);
#8252=EDGE_CURVE('',#6498,#6488,#556,.T.);
#8253=EDGE_CURVE('',#6489,#6498,#557,.T.);
#8254=EDGE_CURVE('',#6495,#6479,#4093,.T.);
#8255=EDGE_CURVE('',#6499,#6497,#4094,.T.);
#8256=EDGE_CURVE('',#6473,#6499,#1347,.T.);
#8257=EDGE_CURVE('',#6477,#6498,#4095,.T.);
#8258=EDGE_CURVE('',#6500,#6494,#1348,.F.);
#8259=EDGE_CURVE('',#6480,#6500,#1349,.F.);
#8260=EDGE_CURVE('',#6501,#6490,#558,.T.);
#8261=EDGE_CURVE('',#6492,#6501,#559,.T.);
#8262=EDGE_CURVE('',#6502,#6487,#98,.T.);
#8263=EDGE_CURVE('',#6503,#6502,#4096,.T.);
#8264=EDGE_CURVE('',#6504,#6503,#99,.T.);
#8265=EDGE_CURVE('',#6505,#6504,#4097,.T.);
#8266=EDGE_CURVE('',#6505,#6476,#4098,.T.);
#8267=EDGE_CURVE('',#6493,#6506,#4099,.T.);
#8268=EDGE_CURVE('',#6507,#6506,#4100,.T.);
#8269=EDGE_CURVE('',#6508,#6507,#100,.T.);
#8270=EDGE_CURVE('',#6509,#6508,#4101,.T.);
#8271=EDGE_CURVE('',#6486,#6509,#101,.T.);
#8272=EDGE_CURVE('',#6494,#6480,#1350,.F.);
#8273=EDGE_CURVE('',#6501,#6496,#4102,.F.);
#8274=EDGE_CURVE('',#6485,#6492,#1351,.T.);
#8275=EDGE_CURVE('',#6510,#6499,#4103,.T.);
#8276=EDGE_CURVE('',#6511,#6510,#1352,.T.);
#8277=EDGE_CURVE('',#6506,#6511,#1353,.T.);
#8278=EDGE_CURVE('',#6512,#6491,#102,.T.);
#8279=EDGE_CURVE('',#6513,#6512,#4104,.T.);
#8280=EDGE_CURVE('',#6514,#6513,#103,.T.);
#8281=EDGE_CURVE('',#6510,#6514,#4105,.T.);
#8282=EDGE_CURVE('',#6515,#6505,#1354,.T.);
#8283=EDGE_CURVE('',#6478,#6515,#4106,.T.);
#8284=EDGE_CURVE('',#6516,#6515,#4107,.T.);
#8285=EDGE_CURVE('',#6517,#6516,#104,.T.);
#8286=EDGE_CURVE('',#6518,#6517,#4108,.T.);
#8287=EDGE_CURVE('',#6483,#6518,#105,.T.);
#8288=EDGE_CURVE('',#6519,#6519,#1355,.T.);
#8289=EDGE_CURVE('',#6519,#6511,#4109,.T.);
#8290=EDGE_CURVE('',#6516,#6514,#1356,.T.);
#8291=EDGE_CURVE('',#6507,#6504,#1357,.T.);
#8292=EDGE_CURVE('',#6518,#6512,#1358,.T.);
#8293=EDGE_CURVE('',#6509,#6502,#1359,.T.);
#8294=EDGE_CURVE('',#6517,#6513,#1360,.T.);
#8295=EDGE_CURVE('',#6508,#6503,#1361,.T.);
#8296=EDGE_CURVE('',#6520,#6520,#1362,.T.);
#8297=EDGE_CURVE('',#6520,#6500,#4110,.T.);
#11187=ORIENTED_EDGE('',*,*,#8209,.F.);
#11188=ORIENTED_EDGE('',*,*,#8210,.T.);
#11189=ORIENTED_EDGE('',*,*,#8211,.T.);
#11190=ORIENTED_EDGE('',*,*,#8212,.T.);
#11191=ORIENTED_EDGE('',*,*,#8213,.F.);
#11192=ORIENTED_EDGE('',*,*,#8214,.T.);
#11193=ORIENTED_EDGE('',*,*,#8209,.T.);
#11194=ORIENTED_EDGE('',*,*,#8215,.T.);
#11195=ORIENTED_EDGE('',*,*,#8216,.F.);
#11196=ORIENTED_EDGE('',*,*,#8217,.T.);
#11197=ORIENTED_EDGE('',*,*,#8218,.F.);
#11198=ORIENTED_EDGE('',*,*,#8219,.F.);
#11199=ORIENTED_EDGE('',*,*,#8220,.F.);
#11200=ORIENTED_EDGE('',*,*,#8221,.F.);
#11201=ORIENTED_EDGE('',*,*,#8222,.T.);
#11202=ORIENTED_EDGE('',*,*,#8216,.T.);
#11203=ORIENTED_EDGE('',*,*,#8223,.F.);
#11204=ORIENTED_EDGE('',*,*,#8224,.F.);
#11205=ORIENTED_EDGE('',*,*,#8225,.F.);
#11206=ORIENTED_EDGE('',*,*,#8226,.F.);
#11207=ORIENTED_EDGE('',*,*,#8227,.T.);
#11208=ORIENTED_EDGE('',*,*,#8223,.T.);
#11209=ORIENTED_EDGE('',*,*,#8219,.T.);
#11210=ORIENTED_EDGE('',*,*,#8228,.F.);
#11211=ORIENTED_EDGE('',*,*,#8229,.F.);
#11212=ORIENTED_EDGE('',*,*,#8215,.F.);
#11213=ORIENTED_EDGE('',*,*,#8212,.F.);
#11214=ORIENTED_EDGE('',*,*,#8230,.F.);
#11215=ORIENTED_EDGE('',*,*,#8231,.F.);
#11216=ORIENTED_EDGE('',*,*,#8232,.T.);
#11217=ORIENTED_EDGE('',*,*,#8233,.F.);
#11218=ORIENTED_EDGE('',*,*,#8234,.T.);
#11219=ORIENTED_EDGE('',*,*,#8235,.T.);
#11220=ORIENTED_EDGE('',*,*,#8236,.F.);
#11221=ORIENTED_EDGE('',*,*,#8237,.T.);
#11222=ORIENTED_EDGE('',*,*,#8238,.F.);
#11223=ORIENTED_EDGE('',*,*,#8239,.T.);
#11224=ORIENTED_EDGE('',*,*,#8240,.T.);
#11225=ORIENTED_EDGE('',*,*,#8231,.T.);
#11226=ORIENTED_EDGE('',*,*,#8241,.F.);
#11227=ORIENTED_EDGE('',*,*,#8242,.T.);
#11228=ORIENTED_EDGE('',*,*,#8243,.T.);
#11229=ORIENTED_EDGE('',*,*,#8244,.F.);
#11230=ORIENTED_EDGE('',*,*,#8210,.F.);
#11231=ORIENTED_EDGE('',*,*,#8214,.F.);
#11232=ORIENTED_EDGE('',*,*,#8245,.F.);
#11233=ORIENTED_EDGE('',*,*,#8246,.F.);
#11234=ORIENTED_EDGE('',*,*,#8217,.F.);
#11235=ORIENTED_EDGE('',*,*,#8222,.F.);
#11236=ORIENTED_EDGE('',*,*,#8247,.F.);
#11237=ORIENTED_EDGE('',*,*,#8248,.F.);
#11238=ORIENTED_EDGE('',*,*,#8235,.F.);
#11239=ORIENTED_EDGE('',*,*,#8249,.F.);
#11240=ORIENTED_EDGE('',*,*,#8250,.F.);
#11241=ORIENTED_EDGE('',*,*,#8251,.F.);
#11242=ORIENTED_EDGE('',*,*,#8252,.F.);
#11243=ORIENTED_EDGE('',*,*,#8253,.F.);
#11244=ORIENTED_EDGE('',*,*,#8239,.F.);
#11245=ORIENTED_EDGE('',*,*,#8220,.T.);
#11246=ORIENTED_EDGE('',*,*,#8227,.F.);
#11247=ORIENTED_EDGE('',*,*,#8254,.F.);
#11248=ORIENTED_EDGE('',*,*,#8251,.T.);
#11249=ORIENTED_EDGE('',*,*,#8255,.F.);
#11250=ORIENTED_EDGE('',*,*,#8256,.F.);
#11251=ORIENTED_EDGE('',*,*,#8257,.F.);
#11252=ORIENTED_EDGE('',*,*,#8232,.F.);
#11253=ORIENTED_EDGE('',*,*,#8240,.F.);
#11254=ORIENTED_EDGE('',*,*,#8253,.T.);
#11255=ORIENTED_EDGE('',*,*,#8218,.T.);
#11256=ORIENTED_EDGE('',*,*,#8246,.T.);
#11257=ORIENTED_EDGE('',*,*,#8258,.F.);
#11258=ORIENTED_EDGE('',*,*,#8259,.F.);
#11259=ORIENTED_EDGE('',*,*,#8228,.T.);
#11260=ORIENTED_EDGE('',*,*,#8260,.F.);
#11261=ORIENTED_EDGE('',*,*,#8261,.F.);
#11262=ORIENTED_EDGE('',*,*,#8242,.F.);
#11263=ORIENTED_EDGE('',*,*,#8224,.T.);
#11264=ORIENTED_EDGE('',*,*,#8257,.T.);
#11265=ORIENTED_EDGE('',*,*,#8252,.T.);
#11266=ORIENTED_EDGE('',*,*,#8238,.T.);
#11267=ORIENTED_EDGE('',*,*,#8262,.F.);
#11268=ORIENTED_EDGE('',*,*,#8263,.F.);
#11269=ORIENTED_EDGE('',*,*,#8264,.F.);
#11270=ORIENTED_EDGE('',*,*,#8265,.F.);
#11271=ORIENTED_EDGE('',*,*,#8266,.T.);
#11272=ORIENTED_EDGE('',*,*,#8236,.T.);
#11273=ORIENTED_EDGE('',*,*,#8230,.T.);
#11274=ORIENTED_EDGE('',*,*,#8211,.F.);
#11275=ORIENTED_EDGE('',*,*,#8244,.T.);
#11276=ORIENTED_EDGE('',*,*,#8267,.T.);
#11277=ORIENTED_EDGE('',*,*,#8268,.F.);
#11278=ORIENTED_EDGE('',*,*,#8269,.F.);
#11279=ORIENTED_EDGE('',*,*,#8270,.F.);
#11280=ORIENTED_EDGE('',*,*,#8271,.F.);
#11281=ORIENTED_EDGE('',*,*,#8213,.T.);
#11282=ORIENTED_EDGE('',*,*,#8229,.T.);
#11283=ORIENTED_EDGE('',*,*,#8272,.F.);
#11284=ORIENTED_EDGE('',*,*,#8245,.T.);
#11285=ORIENTED_EDGE('',*,*,#8261,.T.);
#11286=ORIENTED_EDGE('',*,*,#8273,.T.);
#11287=ORIENTED_EDGE('',*,*,#8249,.T.);
#11288=ORIENTED_EDGE('',*,*,#8274,.T.);
#11289=ORIENTED_EDGE('',*,*,#8247,.T.);
#11290=ORIENTED_EDGE('',*,*,#8221,.T.);
#11291=ORIENTED_EDGE('',*,*,#8256,.T.);
#11292=ORIENTED_EDGE('',*,*,#8275,.F.);
#11293=ORIENTED_EDGE('',*,*,#8276,.F.);
#11294=ORIENTED_EDGE('',*,*,#8277,.F.);
#11295=ORIENTED_EDGE('',*,*,#8267,.F.);
#11296=ORIENTED_EDGE('',*,*,#8260,.T.);
#11297=ORIENTED_EDGE('',*,*,#8241,.T.);
#11298=ORIENTED_EDGE('',*,*,#8278,.F.);
#11299=ORIENTED_EDGE('',*,*,#8279,.F.);
#11300=ORIENTED_EDGE('',*,*,#8280,.F.);
#11301=ORIENTED_EDGE('',*,*,#8281,.F.);
#11302=ORIENTED_EDGE('',*,*,#8275,.T.);
#11303=ORIENTED_EDGE('',*,*,#8255,.T.);
#11304=ORIENTED_EDGE('',*,*,#8250,.T.);
#11305=ORIENTED_EDGE('',*,*,#8273,.F.);
#11306=ORIENTED_EDGE('',*,*,#8225,.T.);
#11307=ORIENTED_EDGE('',*,*,#8266,.F.);
#11308=ORIENTED_EDGE('',*,*,#8282,.F.);
#11309=ORIENTED_EDGE('',*,*,#8283,.F.);
#11310=ORIENTED_EDGE('',*,*,#8226,.T.);
#11311=ORIENTED_EDGE('',*,*,#8283,.T.);
#11312=ORIENTED_EDGE('',*,*,#8284,.F.);
#11313=ORIENTED_EDGE('',*,*,#8285,.F.);
#11314=ORIENTED_EDGE('',*,*,#8286,.F.);
#11315=ORIENTED_EDGE('',*,*,#8287,.F.);
#11316=ORIENTED_EDGE('',*,*,#8233,.T.);
#11317=ORIENTED_EDGE('',*,*,#8248,.T.);
#11318=ORIENTED_EDGE('',*,*,#8254,.T.);
#11319=ORIENTED_EDGE('',*,*,#8288,.T.);
#11320=ORIENTED_EDGE('',*,*,#8289,.T.);
#11321=ORIENTED_EDGE('',*,*,#8276,.T.);
#11322=ORIENTED_EDGE('',*,*,#8281,.T.);
#11323=ORIENTED_EDGE('',*,*,#8290,.F.);
#11324=ORIENTED_EDGE('',*,*,#8284,.T.);
#11325=ORIENTED_EDGE('',*,*,#8282,.T.);
#11326=ORIENTED_EDGE('',*,*,#8265,.T.);
#11327=ORIENTED_EDGE('',*,*,#8291,.F.);
#11328=ORIENTED_EDGE('',*,*,#8268,.T.);
#11329=ORIENTED_EDGE('',*,*,#8277,.T.);
#11330=ORIENTED_EDGE('',*,*,#8289,.F.);
#11331=ORIENTED_EDGE('',*,*,#8278,.T.);
#11332=ORIENTED_EDGE('',*,*,#8243,.F.);
#11333=ORIENTED_EDGE('',*,*,#8274,.F.);
#11334=ORIENTED_EDGE('',*,*,#8234,.F.);
#11335=ORIENTED_EDGE('',*,*,#8287,.T.);
#11336=ORIENTED_EDGE('',*,*,#8292,.T.);
#11337=ORIENTED_EDGE('',*,*,#8271,.T.);
#11338=ORIENTED_EDGE('',*,*,#8293,.T.);
#11339=ORIENTED_EDGE('',*,*,#8262,.T.);
#11340=ORIENTED_EDGE('',*,*,#8237,.F.);
#11341=ORIENTED_EDGE('',*,*,#8279,.T.);
#11342=ORIENTED_EDGE('',*,*,#8292,.F.);
#11343=ORIENTED_EDGE('',*,*,#8286,.T.);
#11344=ORIENTED_EDGE('',*,*,#8294,.T.);
#11345=ORIENTED_EDGE('',*,*,#8270,.T.);
#11346=ORIENTED_EDGE('',*,*,#8295,.T.);
#11347=ORIENTED_EDGE('',*,*,#8263,.T.);
#11348=ORIENTED_EDGE('',*,*,#8293,.F.);
#11349=ORIENTED_EDGE('',*,*,#8280,.T.);
#11350=ORIENTED_EDGE('',*,*,#8294,.F.);
#11351=ORIENTED_EDGE('',*,*,#8285,.T.);
#11352=ORIENTED_EDGE('',*,*,#8290,.T.);
#11353=ORIENTED_EDGE('',*,*,#8269,.T.);
#11354=ORIENTED_EDGE('',*,*,#8291,.T.);
#11355=ORIENTED_EDGE('',*,*,#8264,.T.);
#11356=ORIENTED_EDGE('',*,*,#8295,.F.);
#11357=ORIENTED_EDGE('',*,*,#8296,.F.);
#11358=ORIENTED_EDGE('',*,*,#8297,.T.);
#11359=ORIENTED_EDGE('',*,*,#8258,.T.);
#11360=ORIENTED_EDGE('',*,*,#8272,.T.);
#11361=ORIENTED_EDGE('',*,*,#8259,.T.);
#11362=ORIENTED_EDGE('',*,*,#8297,.F.);
#11363=ORIENTED_EDGE('',*,*,#8296,.T.);
#11364=ORIENTED_EDGE('',*,*,#8288,.F.);
#14952=PLANE('',#16791);
#14953=PLANE('',#16793);
#14954=PLANE('',#16796);
#14955=PLANE('',#16801);
#14956=PLANE('',#16804);
#14957=PLANE('',#16805);
#14958=PLANE('',#16810);
#14959=PLANE('',#16813);
#14960=PLANE('',#16814);
#14961=PLANE('',#16816);
#14962=PLANE('',#16825);
#14963=PLANE('',#16827);
#14964=PLANE('',#16833);
#15558=ADVANCED_FACE('',(#2015),#907,.T.);
#15559=ADVANCED_FACE('',(#2016),#908,.T.);
#15560=ADVANCED_FACE('',(#2017),#909,.T.);
#15561=ADVANCED_FACE('',(#2018),#910,.T.);
#15562=ADVANCED_FACE('',(#2019),#492,.F.);
#15563=ADVANCED_FACE('',(#2020),#14952,.F.);
#15564=ADVANCED_FACE('',(#2021),#14953,.F.);
#15565=ADVANCED_FACE('',(#2022),#14954,.F.);
#15566=ADVANCED_FACE('',(#2023),#493,.F.);
#15567=ADVANCED_FACE('',(#2024),#494,.F.);
#15568=ADVANCED_FACE('',(#2025),#495,.F.);
#15569=ADVANCED_FACE('',(#2026),#911,.T.);
#15570=ADVANCED_FACE('',(#2027),#912,.T.);
#15571=ADVANCED_FACE('',(#2028),#14955,.T.);
#15572=ADVANCED_FACE('',(#2029),#496,.F.);
#15573=ADVANCED_FACE('',(#2030),#14956,.F.);
#15574=ADVANCED_FACE('',(#2031),#14957,.F.);
#15575=ADVANCED_FACE('',(#2032),#913,.T.);
#15576=ADVANCED_FACE('',(#2033),#914,.T.);
#15577=ADVANCED_FACE('',(#2034),#14958,.F.);
#15578=ADVANCED_FACE('',(#2035),#14959,.F.);
#15579=ADVANCED_FACE('',(#2036),#14960,.F.);
#15580=ADVANCED_FACE('',(#2037),#14961,.F.);
#15581=ADVANCED_FACE('',(#2038),#915,.F.);
#15582=ADVANCED_FACE('',(#2039),#1735,.T.);
#15583=ADVANCED_FACE('',(#2040),#1736,.T.);
#15584=ADVANCED_FACE('',(#2041),#14962,.T.);
#15585=ADVANCED_FACE('',(#2042),#14963,.T.);
#15586=ADVANCED_FACE('',(#2043),#1737,.F.);
#15587=ADVANCED_FACE('',(#2044),#1738,.F.);
#15588=ADVANCED_FACE('',(#2045),#1739,.T.);
#15589=ADVANCED_FACE('',(#2046,#1185),#14964,.T.);
#16239=CLOSED_SHELL('',(#15558,#15559,#15560,#15561,#15562,#15563,#15564,
#15565,#15566,#15567,#15568,#15569,#15570,#15571,#15572,#15573,#15574,#15575,
#15576,#15577,#15578,#15579,#15580,#15581,#15582,#15583,#15584,#15585,#15586,
#15587,#15588,#15589));
#16784=AXIS2_PLACEMENT_3D('',#23405,#18997,#18998);
#16785=AXIS2_PLACEMENT_3D('',#23406,#18999,#19000);
#16786=AXIS2_PLACEMENT_3D('',#23499,#19003,#19004);
#16787=AXIS2_PLACEMENT_3D('',#23589,#19006,#19007);
#16788=AXIS2_PLACEMENT_3D('',#23609,#19009,#19010);
#16789=AXIS2_PLACEMENT_3D('',#23621,#19011,#19012);
#16790=AXIS2_PLACEMENT_3D('',#23626,#19014,#19015);
#16791=AXIS2_PLACEMENT_3D('',#23990,#19016,#19017);
#16792=AXIS2_PLACEMENT_3D('',#23995,#19019,#19020);
#16793=AXIS2_PLACEMENT_3D('',#24039,#19021,#19022);
#16794=AXIS2_PLACEMENT_3D('',#24043,#19024,#19025);
#16795=AXIS2_PLACEMENT_3D('',#24081,#19027,#19028);
#16796=AXIS2_PLACEMENT_3D('',#24082,#19029,#19030);
#16797=AXIS2_PLACEMENT_3D('',#24121,#19032,#19033);
#16798=AXIS2_PLACEMENT_3D('',#24448,#19034,#19035);
#16799=AXIS2_PLACEMENT_3D('',#24452,#19038,#19039);
#16800=AXIS2_PLACEMENT_3D('',#24453,#19040,#19041);
#16801=AXIS2_PLACEMENT_3D('',#24455,#19043,#19044);
#16802=AXIS2_PLACEMENT_3D('',#24457,#19045,#19046);
#16803=AXIS2_PLACEMENT_3D('',#24458,#19047,#19048);
#16804=AXIS2_PLACEMENT_3D('',#24493,#19049,#19050);
#16805=AXIS2_PLACEMENT_3D('',#24507,#19054,#19055);
#16806=AXIS2_PLACEMENT_3D('',#24521,#19059,#19060);
#16807=AXIS2_PLACEMENT_3D('',#24522,#19061,#19062);
#16808=AXIS2_PLACEMENT_3D('',#24523,#19063,#19064);
#16809=AXIS2_PLACEMENT_3D('',#24525,#19066,#19067);
#16810=AXIS2_PLACEMENT_3D('',#24526,#19068,#19069);
#16811=AXIS2_PLACEMENT_3D('',#24530,#19071,#19072);
#16812=AXIS2_PLACEMENT_3D('',#24531,#19073,#19074);
#16813=AXIS2_PLACEMENT_3D('',#24532,#19075,#19076);
#16814=AXIS2_PLACEMENT_3D('',#24544,#19079,#19080);
#16815=AXIS2_PLACEMENT_3D('',#24546,#19081,#19082);
#16816=AXIS2_PLACEMENT_3D('',#24548,#19084,#19085);
#16817=AXIS2_PLACEMENT_3D('',#24560,#19088,#19089);
#16818=AXIS2_PLACEMENT_3D('',#24562,#19090,#19091);
#16819=AXIS2_PLACEMENT_3D('',#24564,#19093,#19094);
#16820=AXIS2_PLACEMENT_3D('',#24565,#19095,#19096);
#16821=AXIS2_PLACEMENT_3D('',#24566,#19097,#19098);
#16822=AXIS2_PLACEMENT_3D('',#24567,#19099,#19100);
#16823=AXIS2_PLACEMENT_3D('',#24568,#19101,#19102);
#16824=AXIS2_PLACEMENT_3D('',#24569,#19103,#19104);
#16825=AXIS2_PLACEMENT_3D('',#24570,#19105,#19106);
#16826=AXIS2_PLACEMENT_3D('',#24571,#19107,#19108);
#16827=AXIS2_PLACEMENT_3D('',#24572,#19109,#19110);
#16828=AXIS2_PLACEMENT_3D('',#24573,#19111,#19112);
#16829=AXIS2_PLACEMENT_3D('',#24574,#19113,#19114);
#16830=AXIS2_PLACEMENT_3D('',#24575,#19115,#19116);
#16831=AXIS2_PLACEMENT_3D('',#24576,#19117,#19118);
#16832=AXIS2_PLACEMENT_3D('',#24578,#19119,#19120);
#16833=AXIS2_PLACEMENT_3D('',#24580,#19122,#19123);
#18997=DIRECTION('axis',(0.,0.,1.));
#18998=DIRECTION('refdir',(1.,0.,0.));
#18999=DIRECTION('center_axis',(0.,-1.,0.));
#19000=DIRECTION('ref_axis',(1.,0.,0.));
#19001=DIRECTION('',(0.,1.,0.));
#19002=DIRECTION('',(0.,-1.,0.));
#19003=DIRECTION('center_axis',(0.,-1.,0.));
#19004=DIRECTION('ref_axis',(1.,0.,0.));
#19005=DIRECTION('',(0.,1.,0.));
#19006=DIRECTION('center_axis',(0.,-1.,0.));
#19007=DIRECTION('ref_axis',(0.738759972569494,1.07840993164173E-17,-0.673968621620562));
#19008=DIRECTION('',(0.,-1.,0.));
#19009=DIRECTION('center_axis',(0.,-1.,0.));
#19010=DIRECTION('ref_axis',(1.,1.07840993164173E-17,0.));
#19011=DIRECTION('center_axis',(0.,-1.,0.));
#19012=DIRECTION('ref_axis',(1.,1.07840993164173E-17,0.));
#19013=DIRECTION('',(0.,-1.,0.));
#19014=DIRECTION('center_axis',(0.,1.,0.));
#19015=DIRECTION('ref_axis',(1.,1.07840993164173E-17,0.));
#19016=DIRECTION('center_axis',(0.,1.,0.));
#19017=DIRECTION('ref_axis',(0.,0.,1.));
#19018=DIRECTION('',(-1.,0.,0.));
#19019=DIRECTION('center_axis',(0.,-1.,0.));
#19020=DIRECTION('ref_axis',(1.,0.,0.));
#19021=DIRECTION('center_axis',(0.,1.,0.));
#19022=DIRECTION('ref_axis',(0.,0.,1.));
#19023=DIRECTION('',(1.,0.,0.));
#19024=DIRECTION('center_axis',(0.,-1.,0.));
#19025=DIRECTION('ref_axis',(1.,0.,0.));
#19026=DIRECTION('',(1.,0.,0.));
#19027=DIRECTION('center_axis',(0.,1.,0.));
#19028=DIRECTION('ref_axis',(1.,1.07840993164173E-17,0.));
#19029=DIRECTION('center_axis',(0.,1.,0.));
#19030=DIRECTION('ref_axis',(0.,0.,1.));
#19031=DIRECTION('',(-1.,0.,0.));
#19032=DIRECTION('center_axis',(0.,-1.,0.));
#19033=DIRECTION('ref_axis',(1.,0.,0.));
#19034=DIRECTION('center_axis',(0.,-1.,0.));
#19035=DIRECTION('ref_axis',(1.,1.07840993164173E-17,0.));
#19036=DIRECTION('',(0.,-1.,0.));
#19037=DIRECTION('',(0.,1.,0.));
#19038=DIRECTION('center_axis',(0.,1.,0.));
#19039=DIRECTION('ref_axis',(1.,1.07840993164173E-17,0.));
#19040=DIRECTION('center_axis',(0.,-1.,0.));
#19041=DIRECTION('ref_axis',(1.,1.07840993164173E-17,0.));
#19042=DIRECTION('',(0.,1.,0.));
#19043=DIRECTION('center_axis',(0.,1.,0.));
#19044=DIRECTION('ref_axis',(0.,0.,1.));
#19045=DIRECTION('center_axis',(0.,1.,0.));
#19046=DIRECTION('ref_axis',(1.,0.,0.));
#19047=DIRECTION('center_axis',(0.,1.,0.));
#19048=DIRECTION('ref_axis',(1.,0.,0.));
#19049=DIRECTION('center_axis',(0.,0.,-1.));
#19050=DIRECTION('ref_axis',(1.,0.,0.));
#19051=DIRECTION('',(1.,0.,0.));
#19052=DIRECTION('',(0.,1.,0.));
#19053=DIRECTION('',(1.,0.,0.));
#19054=DIRECTION('center_axis',(0.,0.,-1.));
#19055=DIRECTION('ref_axis',(1.,0.,0.));
#19056=DIRECTION('',(1.,0.,0.));
#19057=DIRECTION('',(0.,-1.,0.));
#19058=DIRECTION('',(1.,0.,0.));
#19059=DIRECTION('center_axis',(0.,-1.,0.));
#19060=DIRECTION('ref_axis',(-0.736568605701436,0.,-0.676362838345694));
#19061=DIRECTION('center_axis',(0.,1.,0.));
#19062=DIRECTION('ref_axis',(1.,0.,0.));
#19063=DIRECTION('center_axis',(0.,-1.,0.));
#19064=DIRECTION('ref_axis',(1.,0.,0.));
#19065=DIRECTION('',(0.,1.,0.));
#19066=DIRECTION('center_axis',(0.,-1.,0.));
#19067=DIRECTION('ref_axis',(1.,0.,0.));
#19068=DIRECTION('center_axis',(0.,-1.,0.));
#19069=DIRECTION('ref_axis',(0.,0.,-1.));
#19070=DIRECTION('',(-1.,0.,0.));
#19071=DIRECTION('center_axis',(0.,1.,0.));
#19072=DIRECTION('ref_axis',(1.,0.,0.));
#19073=DIRECTION('center_axis',(0.,1.,0.));
#19074=DIRECTION('ref_axis',(1.,0.,0.));
#19075=DIRECTION('center_axis',(0.,0.,1.));
#19076=DIRECTION('ref_axis',(-1.,0.,0.));
#19077=DIRECTION('',(-1.,0.,0.));
#19078=DIRECTION('',(0.,1.,0.));
#19079=DIRECTION('center_axis',(0.,-1.,0.));
#19080=DIRECTION('ref_axis',(0.,0.,-1.));
#19081=DIRECTION('center_axis',(0.,1.,0.));
#19082=DIRECTION('ref_axis',(1.,0.,0.));
#19083=DIRECTION('',(-1.,0.,0.));
#19084=DIRECTION('center_axis',(0.,0.,1.));
#19085=DIRECTION('ref_axis',(-1.,0.,0.));
#19086=DIRECTION('',(0.,-1.,0.));
#19087=DIRECTION('',(-1.,0.,0.));
#19088=DIRECTION('center_axis',(0.,-1.,0.));
#19089=DIRECTION('ref_axis',(1.,0.,0.));
#19090=DIRECTION('center_axis',(0.,-1.,0.));
#19091=DIRECTION('ref_axis',(1.,0.,0.));
#19092=DIRECTION('',(0.,1.,0.));
#19093=DIRECTION('center_axis',(0.,-1.,0.));
#19094=DIRECTION('ref_axis',(1.,0.,0.));
#19095=DIRECTION('center_axis',(0.,-1.,0.));
#19096=DIRECTION('ref_axis',(1.,0.,0.));
#19097=DIRECTION('center_axis',(0.,-1.,0.));
#19098=DIRECTION('ref_axis',(1.,0.,0.));
#19099=DIRECTION('center_axis',(0.,-1.,0.));
#19100=DIRECTION('ref_axis',(1.,0.,0.));
#19101=DIRECTION('center_axis',(0.,-1.,0.));
#19102=DIRECTION('ref_axis',(1.,0.,0.));
#19103=DIRECTION('center_axis',(0.,-1.,0.));
#19104=DIRECTION('ref_axis',(1.,0.,0.));
#19105=DIRECTION('center_axis',(0.,1.,0.));
#19106=DIRECTION('ref_axis',(0.,0.,1.));
#19107=DIRECTION('center_axis',(0.,-1.,0.));
#19108=DIRECTION('ref_axis',(1.,0.,0.));
#19109=DIRECTION('center_axis',(0.,1.,0.));
#19110=DIRECTION('ref_axis',(0.,0.,1.));
#19111=DIRECTION('center_axis',(0.,-1.,0.));
#19112=DIRECTION('ref_axis',(1.,0.,0.));
#19113=DIRECTION('center_axis',(0.,1.,0.));
#19114=DIRECTION('ref_axis',(1.,0.,0.));
#19115=DIRECTION('center_axis',(0.,1.,0.));
#19116=DIRECTION('ref_axis',(1.,0.,0.));
#19117=DIRECTION('center_axis',(0.,1.,0.));
#19118=DIRECTION('ref_axis',(1.,0.,0.));
#19119=DIRECTION('center_axis',(0.,-1.,0.));
#19120=DIRECTION('ref_axis',(1.,0.,0.));
#19121=DIRECTION('',(-0.707106781186548,0.707106781186548,-8.65956056235493E-17));
#19122=DIRECTION('center_axis',(0.,-1.,0.));
#19123=DIRECTION('ref_axis',(0.,0.,-1.));
#23405=CARTESIAN_POINT('',(0.,0.,0.));
#23406=CARTESIAN_POINT('Origin',(-0.4,-0.255,9.7));
#23407=CARTESIAN_POINT('',(-1.74415870087061,-0.266244406628447,9.70002284206962));
#23408=CARTESIAN_POINT('',(-1.74424829702886,-0.252155593372042,9.70002193782831));
#23409=CARTESIAN_POINT('',(-1.7442,-0.255,9.7));
#23410=CARTESIAN_POINT('',(-1.74047515456274,-0.167429513866972,9.6));
#23411=CARTESIAN_POINT('Ctrl Pts',(-1.74415870087061,-0.266244406628447,
9.70002284206962));
#23412=CARTESIAN_POINT('Ctrl Pts',(-1.74420569602547,-0.265459972719924,
9.76628025589696));
#23413=CARTESIAN_POINT('Ctrl Pts',(-1.73938151386138,-0.264675538811401,
9.83253088537814));
#23414=CARTESIAN_POINT('Ctrl Pts',(-1.72962299494269,-0.263891104902878,
9.89804654821063));
#23415=CARTESIAN_POINT('Ctrl Pts',(-1.69868589188987,-0.261404240567386,
10.1057486420951));
#23416=CARTESIAN_POINT('Ctrl Pts',(-1.61815580299121,-0.258917376231894,
10.306063888989));
#23417=CARTESIAN_POINT('Ctrl Pts',(-1.49671968419857,-0.256430511896403,
10.4773838643973));
#23418=CARTESIAN_POINT('Ctrl Pts',(-1.37528356540594,-0.253943647560911,
10.6487038398057));
#23419=CARTESIAN_POINT('Ctrl Pts',(-1.21294141671933,-0.25145678322542,
10.7910285437285));
#23420=CARTESIAN_POINT('Ctrl Pts',(-1.02720542034702,-0.248969918889928,
10.8890050939007));
#23421=CARTESIAN_POINT('Ctrl Pts',(-0.841469423974722,-0.246483054554436,
10.9869816440729));
#23422=CARTESIAN_POINT('Ctrl Pts',(-0.632339579916726,-0.243996190218945,
11.0406100404945));
#23423=CARTESIAN_POINT('Ctrl Pts',(-0.422375189109452,-0.241509325883453,
11.0441053064551));
#23424=CARTESIAN_POINT('Ctrl Pts',(-0.212410798302177,-0.239022461547962,
11.0476005724156));
#23425=CARTESIAN_POINT('Ctrl Pts',(-0.00161186074562417,-0.23653559721247,
11.000962707915));
#23426=CARTESIAN_POINT('Ctrl Pts',(0.187282340796658,-0.234048732876978,
10.9092225683747));
#23427=CARTESIAN_POINT('Ctrl Pts',(0.37617654233894,-0.231561868541487,
10.8174824288345));
#23428=CARTESIAN_POINT('Ctrl Pts',(0.543166007866952,-0.229075004205995,
10.6806400142546));
#23429=CARTESIAN_POINT('Ctrl Pts',(0.670237130981439,-0.226588139870503,
10.5134569577609));
#23430=CARTESIAN_POINT('Ctrl Pts',(0.797308254095925,-0.224101275535012,
10.3462739012672));
#23431=CARTESIAN_POINT('Ctrl Pts',(0.884461034796888,-0.22161441119952,
10.1487502028598));
#23432=CARTESIAN_POINT('Ctrl Pts',(0.9222943334795,-0.219127546864029,9.94219283449699));
#23433=CARTESIAN_POINT('Ctrl Pts',(0.960127632162113,-0.216640682528537,
9.73563546613418));
#23434=CARTESIAN_POINT('Ctrl Pts',(0.948641448826376,-0.214153818193045,
9.52004442781599));
#23435=CARTESIAN_POINT('Ctrl Pts',(0.889074364684035,-0.211666953857554,
9.31867669316543));
#23436=CARTESIAN_POINT('Ctrl Pts',(0.829507280541693,-0.209180089522062,
9.11730895851487));
#23437=CARTESIAN_POINT('Ctrl Pts',(0.721859295592745,-0.206693225186571,
8.93016452753194));
#23438=CARTESIAN_POINT('Ctrl Pts',(0.577743655398177,-0.204206360851079,
8.77742952694693));
#23439=CARTESIAN_POINT('Ctrl Pts',(0.43362801520361,-0.201719496515587,
8.62469452636193));
#23440=CARTESIAN_POINT('Ctrl Pts',(0.253044719763425,-0.199232632180096,
8.50636895617486));
#23441=CARTESIAN_POINT('Ctrl Pts',(0.0554715964079175,-0.196745767844604,
8.43522018029139));
#23442=CARTESIAN_POINT('Ctrl Pts',(-0.142101526947592,-0.194258903509113,
8.36407140440791));
#23443=CARTESIAN_POINT('Ctrl Pts',(-0.356664478218423,-0.191772039173621,
8.34009942282803));
#23444=CARTESIAN_POINT('Ctrl Pts',(-0.565066781035095,-0.189285174838129,
8.36588291802197));
#23445=CARTESIAN_POINT('Ctrl Pts',(-0.773469083851767,-0.186798310502638,
8.39166641321591));
#23446=CARTESIAN_POINT('Ctrl Pts',(-0.975710738214278,-0.184311446167146,
8.46720538518367));
#23447=CARTESIAN_POINT('Ctrl Pts',(-1.14998417762288,-0.181824581831655,
8.58436696040311));
#23448=CARTESIAN_POINT('Ctrl Pts',(-1.32425761703147,-0.179337717496163,
8.70152853562254));
#23449=CARTESIAN_POINT('Ctrl Pts',(-1.47056284148616,-0.176850853160671,
8.86031271409366));
#23450=CARTESIAN_POINT('Ctrl Pts',(-1.57308686213316,-0.17436398882518,
9.04355598262635));
#23451=CARTESIAN_POINT('Ctrl Pts',(-1.66838092966563,-0.172052497172444,
9.21387700882323));
#23452=CARTESIAN_POINT('Ctrl Pts',(-1.72585093496104,-0.169741005519708,
9.40532906990018));
#23453=CARTESIAN_POINT('Ctrl Pts',(-1.74046409013886,-0.167429513866973,
9.6000014831431));
#23454=CARTESIAN_POINT('',(-1.74047515456274,-0.153340700610567,9.6));
#23455=CARTESIAN_POINT('',(-1.74047515456274,-0.255,9.6));
#23456=CARTESIAN_POINT('Ctrl Pts',(-1.74047515456274,-0.153340700610567,
9.6));
#23457=CARTESIAN_POINT('Ctrl Pts',(-1.72473294771491,-0.155846150645574,
9.38897962842498));
#23458=CARTESIAN_POINT('Ctrl Pts',(-1.65828106796239,-0.158351600680581,
9.18182683781037));
#23459=CARTESIAN_POINT('Ctrl Pts',(-1.54831356305132,-0.160857050715588,
9.00111449525873));
#23460=CARTESIAN_POINT('Ctrl Pts',(-1.43834605814026,-0.163362500750596,
8.82040215270709));
#23461=CARTESIAN_POINT('Ctrl Pts',(-1.28486292807066,-0.165867950785603,
8.66613025821842));
#23462=CARTESIAN_POINT('Ctrl Pts',(-1.10470058034043,-0.16837340082061,
8.55522077011294));
#23463=CARTESIAN_POINT('Ctrl Pts',(-0.924538232610208,-0.170878850855617,
8.44431128200746));
#23464=CARTESIAN_POINT('Ctrl Pts',(-0.717696667219359,-0.173384300890624,
8.37676420028517));
#23465=CARTESIAN_POINT('Ctrl Pts',(-0.506806067411535,-0.175889750925631,
8.3599572690053));
#23466=CARTESIAN_POINT('Ctrl Pts',(-0.295915467603711,-0.178395200960638,
8.34315033772542));
#23467=CARTESIAN_POINT('Ctrl Pts',(-0.0809758333789124,-0.180900650995646,
8.37708355688795));
#23468=CARTESIAN_POINT('Ctrl Pts',(0.114479473573055,-0.183406101030653,
8.45804996515167));
#23469=CARTESIAN_POINT('Ctrl Pts',(0.309934780525024,-0.18591155106566,
8.53901637341539));
#23470=CARTESIAN_POINT('Ctrl Pts',(0.485905760204162,-0.188417001100667,
8.66701597078031));
#23471=CARTESIAN_POINT('Ctrl Pts',(0.6231331327789,-0.190922451135674,8.82803444612455));
#23472=CARTESIAN_POINT('Ctrl Pts',(0.760360505353638,-0.193427901170681,
8.9890529214688));
#23473=CARTESIAN_POINT('Ctrl Pts',(0.858844270823975,-0.195933351205688,
9.18309027479239));
#23474=CARTESIAN_POINT('Ctrl Pts',(0.907803125803339,-0.198438801240696,
9.38890870639347));
#23475=CARTESIAN_POINT('Ctrl Pts',(0.956761980782702,-0.200944251275703,
9.59472713799455));
#23476=CARTESIAN_POINT('Ctrl Pts',(0.956195925271092,-0.20344970131071,
9.81232664787314));
#23477=CARTESIAN_POINT('Ctrl Pts',(0.90616748485386,-0.205955151345717,
10.0178879803874));
#23478=CARTESIAN_POINT('Ctrl Pts',(0.856139044436628,-0.208460601380724,
10.2234493129017));
#23479=CARTESIAN_POINT('Ctrl Pts',(0.756648219113773,-0.210966051415731,
10.4169724680517));
#23480=CARTESIAN_POINT('Ctrl Pts',(0.618585043209539,-0.213471501450739,
10.5772746807812));
#23481=CARTESIAN_POINT('Ctrl Pts',(0.480521867305305,-0.215976951485746,
10.7375768935107));
#23482=CARTESIAN_POINT('Ctrl Pts',(0.303886340819692,-0.218482401520753,
10.8646581638196));
#23483=CARTESIAN_POINT('Ctrl Pts',(0.108013169915432,-0.22098785155576,
10.9446079735783));
#23484=CARTESIAN_POINT('Ctrl Pts',(-0.0878600009888281,-0.223493301590767,
11.0245577833369));
#23485=CARTESIAN_POINT('Ctrl Pts',(-0.302970816311735,-0.225998751625774,
11.0573761325454));
#23486=CARTESIAN_POINT('Ctrl Pts',(-0.513773231433628,-0.228504201660781,
11.0394707880266));
#23487=CARTESIAN_POINT('Ctrl Pts',(-0.724575646555521,-0.231009651695789,
11.0215654435079));
#23488=CARTESIAN_POINT('Ctrl Pts',(-0.9310696614764,-0.233515101730796,
10.9529364052621));
#23489=CARTESIAN_POINT('Ctrl Pts',(-1.1106523459517,-0.236020551765803,
10.8410957962038));
#23490=CARTESIAN_POINT('Ctrl Pts',(-1.290235030427,-0.23852600180081,10.7292551871455));
#23491=CARTESIAN_POINT('Ctrl Pts',(-1.44290638445672,-0.241031451835817,
10.5742030072748));
#23492=CARTESIAN_POINT('Ctrl Pts',(-1.55195496298315,-0.243536901870824,
10.3929113359787));
#23493=CARTESIAN_POINT('Ctrl Pts',(-1.66100354150958,-0.246042351905831,
10.2116196646827));
#23494=CARTESIAN_POINT('Ctrl Pts',(-1.72642934453273,-0.248547801940839,
10.0040885019612));
#23495=CARTESIAN_POINT('Ctrl Pts',(-1.74107083610881,-0.251053251975846,
9.79303427067891));
#23496=CARTESIAN_POINT('Ctrl Pts',(-1.74321814458179,-0.251420699107911,
9.76208123992141));
#23497=CARTESIAN_POINT('Ctrl Pts',(-1.74427313829983,-0.251788146239977,
9.73105243182909));
#23498=CARTESIAN_POINT('Ctrl Pts',(-1.74424829702886,-0.252155593372042,
9.70002193782831));
#23499=CARTESIAN_POINT('Origin',(-0.4,-0.255,9.7));
#23500=CARTESIAN_POINT('',(-1.74415902867232,-0.366244406628447,9.69997584025059));
#23501=CARTESIAN_POINT('',(-1.74411350535466,-0.352155593372042,9.70000771515446));
#23502=CARTESIAN_POINT('',(-1.7442,-0.255,9.7));
#23503=CARTESIAN_POINT('Ctrl Pts',(-1.74415902867232,-0.366244406628447,
9.69997584025059));
#23504=CARTESIAN_POINT('Ctrl Pts',(-1.74404578241023,-0.364455875747981,
9.85103608154908));
#23505=CARTESIAN_POINT('Ctrl Pts',(-1.7185672270758,-0.362667344867516,
10.0021470613059));
#23506=CARTESIAN_POINT('Ctrl Pts',(-1.66861307355174,-0.36087881398705,
10.1446731556306));
#23507=CARTESIAN_POINT('Ctrl Pts',(-1.59915427685692,-0.358391949651559,
10.342848688815));
#23508=CARTESIAN_POINT('Ctrl Pts',(-1.48237549311787,-0.355905085316067,
10.5244266024324));
#23509=CARTESIAN_POINT('Ctrl Pts',(-1.3308763368522,-0.353418220980575,
10.6698374482951));
#23510=CARTESIAN_POINT('Ctrl Pts',(-1.17937718058652,-0.350931356645084,
10.8152482941577));
#23511=CARTESIAN_POINT('Ctrl Pts',(-0.993157651794214,-0.348444492309592,
10.9244920722656));
#23512=CARTESIAN_POINT('Ctrl Pts',(-0.792305418029019,-0.345957627974101,
10.9857755739092));
#23513=CARTESIAN_POINT('Ctrl Pts',(-0.591453184263824,-0.343470763638609,
11.0470590755528));
#23514=CARTESIAN_POINT('Ctrl Pts',(-0.375968245525741,-0.340983899303117,
11.0603823007321));
#23515=CARTESIAN_POINT('Ctrl Pts',(-0.169095752144418,-0.338497034967626,
11.0243119578645));
#23516=CARTESIAN_POINT('Ctrl Pts',(0.0377767412369071,-0.336010170632134,
10.988241614997));
#23517=CARTESIAN_POINT('Ctrl Pts',(0.236036789261473,-0.333523306296643,
10.9027777040825));
#23518=CARTESIAN_POINT('Ctrl Pts',(0.40429775759656,-0.331036441961151,
10.7771375488516));
#23519=CARTESIAN_POINT('Ctrl Pts',(0.572558725931644,-0.328549577625659,
10.6514973936206));
#23520=CARTESIAN_POINT('Ctrl Pts',(0.71082061457725,-0.326062713290168,
10.4856809940731));
#23521=CARTESIAN_POINT('Ctrl Pts',(0.80416876135257,-0.323575848954676,
10.2975761605154));
#23522=CARTESIAN_POINT('Ctrl Pts',(0.897516908127891,-0.321088984619184,
10.1094713269576));
#23523=CARTESIAN_POINT('Ctrl Pts',(0.945951313032926,-0.318602120283693,
9.8990780593896));
#23524=CARTESIAN_POINT('Ctrl Pts',(0.944247277856241,-0.316115255948201,
9.68909153369745));
#23525=CARTESIAN_POINT('Ctrl Pts',(0.942543242679555,-0.31362839161271,
9.4791050080053));
#23526=CARTESIAN_POINT('Ctrl Pts',(0.890700767421149,-0.311141527277218,
9.26952522418903));
#23527=CARTESIAN_POINT('Ctrl Pts',(0.794312198032813,-0.308654662941726,
9.08296017850674));
#23528=CARTESIAN_POINT('Ctrl Pts',(0.69792362864448,-0.306167798606235,
8.89639513282446));
#23529=CARTESIAN_POINT('Ctrl Pts',(0.556988965126219,-0.303680934270743,
8.73284482527617));
#23530=CARTESIAN_POINT('Ctrl Pts',(0.3867111337889,-0.301194069935252,8.60995169102424));
#23531=CARTESIAN_POINT('Ctrl Pts',(0.216433302451579,-0.29870720559976,
8.48705855677231));
#23532=CARTESIAN_POINT('Ctrl Pts',(0.0168123032952003,-0.296220341264268,
8.40482259581673));
#23533=CARTESIAN_POINT('Ctrl Pts',(-0.190618325459444,-0.293733476928777,
8.37211481407425));
#23534=CARTESIAN_POINT('Ctrl Pts',(-0.398048954214088,-0.291246612593285,
8.33940703233177));
#23535=CARTESIAN_POINT('Ctrl Pts',(-0.613289212566997,-0.288759748257794,
8.35622742980239));
#23536=CARTESIAN_POINT('Ctrl Pts',(-0.813120676364068,-0.286272883922302,
8.42076153704854));
#23537=CARTESIAN_POINT('Ctrl Pts',(-1.01295214016114,-0.28378601958681,
8.48529564429469));
#23538=CARTESIAN_POINT('Ctrl Pts',(-1.19737480940237,-0.281299155251319,
8.59754346131637));
#23539=CARTESIAN_POINT('Ctrl Pts',(-1.34649461965064,-0.278812290915827,
8.7453965855336));
#23540=CARTESIAN_POINT('Ctrl Pts',(-1.4956144298989,-0.276325426580336,
8.89324970975083));
#23541=CARTESIAN_POINT('Ctrl Pts',(-1.6094313811542,-0.273838562244844,
9.0767081411636));
#23542=CARTESIAN_POINT('Ctrl Pts',(-1.67566779817835,-0.271351697909352,
9.27598182730744));
#23543=CARTESIAN_POINT('Ctrl Pts',(-1.72101120115614,-0.269649267482384,
9.41239843103761));
#23544=CARTESIAN_POINT('Ctrl Pts',(-1.74405670887271,-0.267946837055416,
9.55622661387719));
#23545=CARTESIAN_POINT('Ctrl Pts',(-1.74415870087061,-0.266244406628447,
9.70002284206962));
#23546=CARTESIAN_POINT('Ctrl Pts',(-1.74424829702886,-0.252155593372042,
9.70002193782831));
#23547=CARTESIAN_POINT('Ctrl Pts',(-1.74410375729837,-0.254293596274984,
9.51947001494231));
#23548=CARTESIAN_POINT('Ctrl Pts',(-1.70740106403156,-0.256431599177926,
9.33886101509463));
#23549=CARTESIAN_POINT('Ctrl Pts',(-1.63659858427149,-0.258569602080867,
9.17279007747477));
#23550=CARTESIAN_POINT('Ctrl Pts',(-1.55362766072905,-0.261075052115874,
8.97817741539611));
#23551=CARTESIAN_POINT('Ctrl Pts',(-1.42382863351516,-0.263580502150882,
8.80352939108198));
#23552=CARTESIAN_POINT('Ctrl Pts',(-1.26140934623515,-0.266085952185889,
8.6679630339014));
#23553=CARTESIAN_POINT('Ctrl Pts',(-1.09899005895515,-0.268591402220896,
8.53239667672083));
#23554=CARTESIAN_POINT('Ctrl Pts',(-0.903950511609032,-0.271096852255903,
8.43591198667381));
#23555=CARTESIAN_POINT('Ctrl Pts',(-0.697639798691326,-0.27360230229091,
8.38907021096974));
#23556=CARTESIAN_POINT('Ctrl Pts',(-0.49132908577362,-0.276107752325917,
8.34222843526567));
#23557=CARTESIAN_POINT('Ctrl Pts',(-0.273747207284324,-0.278613202360924,
8.34502957390454));
#23558=CARTESIAN_POINT('Ctrl Pts',(-0.0687107480140969,-0.281118652395932,
8.39716701276829));
#23559=CARTESIAN_POINT('Ctrl Pts',(0.136325711256132,-0.283624102430939,
8.44930445163204));
#23560=CARTESIAN_POINT('Ctrl Pts',(0.328816751307292,-0.286129552465946,
8.55077819072068));
#23561=CARTESIAN_POINT('Ctrl Pts',(0.487692238606602,-0.288635002500953,
8.69048088128578));
#23562=CARTESIAN_POINT('Ctrl Pts',(0.646567725905912,-0.29114045253596,
8.83018357185089));
#23563=CARTESIAN_POINT('Ctrl Pts',(0.771827660453372,-0.293645902570967,
9.00811521389247));
#23564=CARTESIAN_POINT('Ctrl Pts',(0.849761047925756,-0.296151352605974,
9.20479934949277));
#23565=CARTESIAN_POINT('Ctrl Pts',(0.927694435398139,-0.298656802640981,
9.40148348509306));
#23566=CARTESIAN_POINT('Ctrl Pts',(0.958301275795446,-0.301162252675989,
9.61692011425207));
#23567=CARTESIAN_POINT('Ctrl Pts',(0.938231334443277,-0.303667702710996,
9.82752747368889));
#23568=CARTESIAN_POINT('Ctrl Pts',(0.918161393091109,-0.306173152746003,
10.0381348331257));
#23569=CARTESIAN_POINT('Ctrl Pts',(0.847414669989466,-0.30867860278101,
10.2439129228403));
#23570=CARTESIAN_POINT('Ctrl Pts',(0.733735124390046,-0.311184052816017,
10.4223372001404));
#23571=CARTESIAN_POINT('Ctrl Pts',(0.620055578790627,-0.313689502851024,
10.6007614774404));
#23572=CARTESIAN_POINT('Ctrl Pts',(0.463443210693432,-0.316194952886031,
10.7518319423259));
#23573=CARTESIAN_POINT('Ctrl Pts',(0.281040863626771,-0.318700402921038,
10.8590123805809));
#23574=CARTESIAN_POINT('Ctrl Pts',(0.0986385165601081,-0.321205852956046,
10.9661928188359));
#23575=CARTESIAN_POINT('Ctrl Pts',(-0.10955380947602,-0.323711302991053,
11.0294832304604));
#23576=CARTESIAN_POINT('Ctrl Pts',(-0.320747316145784,-0.32621675302606,
11.0419558059126));
#23577=CARTESIAN_POINT('Ctrl Pts',(-0.531940822815548,-0.328722203061067,
11.0544283813648));
#23578=CARTESIAN_POINT('Ctrl Pts',(-0.746135510118948,-0.331227653096074,
11.0160831206447));
#23579=CARTESIAN_POINT('Ctrl Pts',(-0.939885549343526,-0.333733103131081,
10.9311173517491));
#23580=CARTESIAN_POINT('Ctrl Pts',(-1.1336355885681,-0.336238553166089,
10.8461515828534));
#23581=CARTESIAN_POINT('Ctrl Pts',(-1.30694097971386,-0.338744003201096,
10.7145653057822));
#23582=CARTESIAN_POINT('Ctrl Pts',(-1.44083167143585,-0.341249453236103,
10.5507619058457));
#23583=CARTESIAN_POINT('Ctrl Pts',(-1.57472236315784,-0.34375490327111,
10.3869585059092));
#23584=CARTESIAN_POINT('Ctrl Pts',(-1.66919835545607,-0.346260353306117,
10.1909379831076));
#23585=CARTESIAN_POINT('Ctrl Pts',(-1.71391824344407,-0.348765803341124,
9.98415700824511));
#23586=CARTESIAN_POINT('Ctrl Pts',(-1.73408641394803,-0.34989573335143,
9.89090109581708));
#23587=CARTESIAN_POINT('Ctrl Pts',(-1.7441346438382,-0.351025663361736,
9.79545660497557));
#23588=CARTESIAN_POINT('Ctrl Pts',(-1.74411350535466,-0.352155593372042,
9.70000771515446));
#23589=CARTESIAN_POINT('Origin',(-0.4,0.0506589891902575,9.7));
#23590=CARTESIAN_POINT('',(-1.68683546212087,-0.299341010809742,9.70002186794253));
#23591=CARTESIAN_POINT('',(-1.68679219402118,-0.319058989190747,9.70000738613257));
#23592=CARTESIAN_POINT('',(-1.686875,0.0506589891902575,9.7));
#23593=CARTESIAN_POINT('',(-0.517805766168008,-0.3758,10.9813944679847));
#23594=CARTESIAN_POINT('Ctrl Pts',(-1.68683546212087,-0.299341010809742,
9.70002186794253));
#23595=CARTESIAN_POINT('Ctrl Pts',(-1.68673781969243,-0.301043441236711,
9.56235800009911));
#23596=CARTESIAN_POINT('Ctrl Pts',(-1.63244651236718,-0.305232735999171,
9.22352319669137));
#23597=CARTESIAN_POINT('Ctrl Pts',(-1.33992756310779,-0.311908895097122,
8.75201990128797));
#23598=CARTESIAN_POINT('Ctrl Pts',(-0.810254324423489,-0.319369488103597,
8.42963727326435));
#23599=CARTESIAN_POINT('Ctrl Pts',(-0.192071076094596,-0.326830081110072,
8.38132805812896));
#23600=CARTESIAN_POINT('Ctrl Pts',(0.381252700031053,-0.334290674116547,
8.61751479132649));
#23601=CARTESIAN_POINT('Ctrl Pts',(0.786025713976292,-0.341751267123022,
9.08724132463895));
#23602=CARTESIAN_POINT('Ctrl Pts',(0.934920488596498,-0.349211860129497,
9.68916734226706));
#23603=CARTESIAN_POINT('Ctrl Pts',(0.795813901454333,-0.356672453135971,
10.2934297352181));
#23604=CARTESIAN_POINT('Ctrl Pts',(0.398717261183206,-0.364133046142446,
10.7696646240018));
#23605=CARTESIAN_POINT('Ctrl Pts',(-0.0879068301996579,-0.370508895097122,
10.9794335532901));
#23606=CARTESIAN_POINT('Ctrl Pts',(-0.404889468122248,-0.374397879716307,
10.9917424685781));
#23607=CARTESIAN_POINT('Ctrl Pts',(-0.517805766168008,-0.3758,10.9813944679847));
#23608=CARTESIAN_POINT('',(0.773161008253381,-0.3758,10.228905014477));
#23609=CARTESIAN_POINT('Origin',(-0.4,-0.3758,9.7));
#23610=CARTESIAN_POINT('Ctrl Pts',(-1.68679219402118,-0.319058989190747,
9.70000738613257));
#23611=CARTESIAN_POINT('Ctrl Pts',(-1.68676755850452,-0.320434509215448,
9.58876796298132));
#23612=CARTESIAN_POINT('Ctrl Pts',(-1.64639120365236,-0.324315479275156,
9.27489314898718));
#23613=CARTESIAN_POINT('Ctrl Pts',(-1.39395194797187,-0.330701899369872,
8.80772380021452));
#23614=CARTESIAN_POINT('Ctrl Pts',(-0.879252204171272,-0.338218249474893,
8.45324089690315));
#23615=CARTESIAN_POINT('Ctrl Pts',(-0.259635570614986,-0.345734599579915,
8.3716914957747));
#23616=CARTESIAN_POINT('Ctrl Pts',(0.329254578046856,-0.353250949684936,
8.58095279849071));
#23617=CARTESIAN_POINT('Ctrl Pts',(0.758488001187141,-0.360767299789957,
9.03515948120896));
#23618=CARTESIAN_POINT('Ctrl Pts',(0.934107096026125,-0.368283649894978,
9.63498649925687));
#23619=CARTESIAN_POINT('Ctrl Pts',(0.856422329660891,-0.373294549964993,
10.0442235818997));
#23620=CARTESIAN_POINT('Ctrl Pts',(0.773161008253379,-0.3758,10.228905014477));
#23621=CARTESIAN_POINT('Origin',(-0.4,0.0506589891902575,9.7));
#23622=CARTESIAN_POINT('',(-1.686875,-0.2,9.7));
#23623=CARTESIAN_POINT('',(-1.6869212373449,-0.219058989190747,9.70002100226366));
#23624=CARTESIAN_POINT('',(-1.686875,0.0506589891902575,9.7));
#23625=CARTESIAN_POINT('',(-1.68577203777491,-0.2,9.64673150554831));
#23626=CARTESIAN_POINT('Origin',(-0.4,-0.2,9.7));
#23627=CARTESIAN_POINT('Ctrl Pts',(-1.68577203777491,-0.2,9.64673150554831));
#23628=CARTESIAN_POINT('Ctrl Pts',(-1.67744860675331,-0.202486864335492,
9.44582410285027));
#23629=CARTESIAN_POINT('Ctrl Pts',(-1.56497328697934,-0.207460593006475,
9.04813481150073));
#23630=CARTESIAN_POINT('Ctrl Pts',(-1.14477569200808,-0.21492118601295,
8.59209689377269));
#23631=CARTESIAN_POINT('Ctrl Pts',(-0.563925233093278,-0.222381779019424,
8.3751443244727));
#23632=CARTESIAN_POINT('Ctrl Pts',(0.0523127476759186,-0.229842372025899,
8.44399332862896));
#23633=CARTESIAN_POINT('Ctrl Pts',(0.570959068877206,-0.237302965032374,
8.78383163721656));
#23634=CARTESIAN_POINT('Ctrl Pts',(0.880130696531965,-0.244763558038849,
9.32132194287307));
#23635=CARTESIAN_POINT('Ctrl Pts',(0.913119720888853,-0.252224151045324,
9.94051265281741));
#23636=CARTESIAN_POINT('Ctrl Pts',(0.662811579247987,-0.259684744051799,
10.5078128523146));
#23637=CARTESIAN_POINT('Ctrl Pts',(0.183207572884291,-0.267145337058273,
10.9008326758436));
#23638=CARTESIAN_POINT('Ctrl Pts',(-0.422219929201908,-0.274605930064748,
11.0347794885482));
#23639=CARTESIAN_POINT('Ctrl Pts',(-1.02285369219581,-0.282066523071223,
10.8807554386038));
#23640=CARTESIAN_POINT('Ctrl Pts',(-1.48911031901715,-0.289527116077698,
10.4719901431999));
#23641=CARTESIAN_POINT('Ctrl Pts',(-1.6676202903207,-0.295285278657204,
10.0279540138011));
#23642=CARTESIAN_POINT('Ctrl Pts',(-1.68688045311172,-0.298556576901219,
9.76345365593468));
#23643=CARTESIAN_POINT('Ctrl Pts',(-1.68683546212087,-0.299341010809742,
9.70002186794253));
#23644=CARTESIAN_POINT('Ctrl Pts',(-1.6869212373449,-0.219058989190747,
9.70002100226366));
#23645=CARTESIAN_POINT('Ctrl Pts',(-1.68678286168229,-0.221196992093688,
9.52716892983104));
#23646=CARTESIAN_POINT('Ctrl Pts',(-1.61046904669073,-0.225840445031637,
9.15163894624125));
#23647=CARTESIAN_POINT('Ctrl Pts',(-1.25590265556386,-0.232989348004593,
8.67456048866193));
#23648=CARTESIAN_POINT('Ctrl Pts',(-0.695737090563785,-0.240505698109614,
8.39745052994095));
#23649=CARTESIAN_POINT('Ctrl Pts',(-0.0708285653125278,-0.248022048214636,
8.40549557223947));
#23650=CARTESIAN_POINT('Ctrl Pts',(0.482017530132723,-0.255538398319657,
8.69693438638102));
#23651=CARTESIAN_POINT('Ctrl Pts',(0.841771759274435,-0.263054748424679,
9.20796499607955));
#23652=CARTESIAN_POINT('Ctrl Pts',(0.929676485661023,-0.2705710985297,9.8267122334304));
#23653=CARTESIAN_POINT('Ctrl Pts',(0.726487549584337,-0.278087448634722,
10.4177195519875));
#23654=CARTESIAN_POINT('Ctrl Pts',(0.276687204706167,-0.285603798739743,
10.8516032102962));
#23655=CARTESIAN_POINT('Ctrl Pts',(-0.321253948919206,-0.293120148844764,
11.0333771616263));
#23656=CARTESIAN_POINT('Ctrl Pts',(-0.936434252944416,-0.300636498949786,
10.923247216553));
#23657=CARTESIAN_POINT('Ctrl Pts',(-1.43417798579078,-0.308152849054807,
10.5453233429344));
#23658=CARTESIAN_POINT('Ctrl Pts',(-1.65586245541949,-0.314293679135128,
10.0853683366248));
#23659=CARTESIAN_POINT('Ctrl Pts',(-1.68681243102907,-0.317929059180441,
9.7913857450736));
#23660=CARTESIAN_POINT('Ctrl Pts',(-1.68679219402118,-0.319058989190747,
9.70000738613257));
#23661=CARTESIAN_POINT('Ctrl Pts',(-1.68330900500515,-0.120244096429272,
9.60426461836037));
#23662=CARTESIAN_POINT('Ctrl Pts',(-1.66823814320088,-0.122749546464279,
9.40224346029563));
#23663=CARTESIAN_POINT('Ctrl Pts',(-1.5410022218253,-0.127760446534293,
9.00560643095153));
#23664=CARTESIAN_POINT('Ctrl Pts',(-1.10018924085152,-0.135276796639315,
8.56252807009725));
#23665=CARTESIAN_POINT('Ctrl Pts',(-0.506127554802531,-0.142793146744336,
8.36852870067744));
#23666=CARTESIAN_POINT('Ctrl Pts',(0.111192282557321,-0.150309496849357,
8.46598699128103));
#23667=CARTESIAN_POINT('Ctrl Pts',(0.616591749469812,-0.157825846954379,
8.83360970038453));
#23668=CARTESIAN_POINT('Ctrl Pts',(0.899443175648149,-0.1653421970594,9.39089690256787));
#23669=CARTESIAN_POINT('Ctrl Pts',(0.897817429435154,-0.172858547164422,
10.0158560662526));
#23670=CARTESIAN_POINT('Ctrl Pts',(0.612073665477375,-0.180374897269443,
10.5716664596844));
#23671=CARTESIAN_POINT('Ctrl Pts',(0.104765579300823,-0.187891247374464,
10.9366516770526));
#23672=CARTESIAN_POINT('Ctrl Pts',(-0.513045900691733,-0.195407597479486,
11.0309079926402));
#23673=CARTESIAN_POINT('Ctrl Pts',(-1.10610940043427,-0.202923947584507,
10.8338011775994));
#23674=CARTESIAN_POINT('Ctrl Pts',(-1.54459091073853,-0.210440297689529,
10.3884817891799));
#23675=CARTESIAN_POINT('Ctrl Pts',(-1.73249783738354,-0.21795664779455,
9.79243953722229));
#23676=CARTESIAN_POINT('Ctrl Pts',(-1.62869343776713,-0.225472997899572,
9.1761603464716));
#23677=CARTESIAN_POINT('Ctrl Pts',(-1.25590265556386,-0.232989348004593,
8.67456048866193));
#23678=CARTESIAN_POINT('Ctrl Pts',(-0.695737090563785,-0.240505698109614,
8.39745052994095));
#23679=CARTESIAN_POINT('Ctrl Pts',(-0.0708285653125278,-0.248022048214636,
8.40549557223947));
#23680=CARTESIAN_POINT('Ctrl Pts',(0.482017530132723,-0.255538398319657,
8.69693438638102));
#23681=CARTESIAN_POINT('Ctrl Pts',(0.841771759274435,-0.263054748424679,
9.20796499607955));
#23682=CARTESIAN_POINT('Ctrl Pts',(0.929676485661023,-0.2705710985297,9.8267122334304));
#23683=CARTESIAN_POINT('Ctrl Pts',(0.726487549584337,-0.278087448634722,
10.4177195519875));
#23684=CARTESIAN_POINT('Ctrl Pts',(0.276687204706167,-0.285603798739743,
10.8516032102962));
#23685=CARTESIAN_POINT('Ctrl Pts',(-0.321253948919206,-0.293120148844764,
11.0333771616263));
#23686=CARTESIAN_POINT('Ctrl Pts',(-0.936434252944416,-0.300636498949786,
10.923247216553));
#23687=CARTESIAN_POINT('Ctrl Pts',(-1.43417798579078,-0.308152849054807,
10.5453233429344));
#23688=CARTESIAN_POINT('Ctrl Pts',(-1.7055188411444,-0.315669199159829,
9.98234035614576));
#23689=CARTESIAN_POINT('Ctrl Pts',(-1.69105451839558,-0.32318554926485,
9.35754801027796));
#23690=CARTESIAN_POINT('Ctrl Pts',(-1.39395194797187,-0.330701899369872,
8.80772380021452));
#23691=CARTESIAN_POINT('Ctrl Pts',(-0.879252204171272,-0.338218249474893,
8.45324089690315));
#23692=CARTESIAN_POINT('Ctrl Pts',(-0.259635570614986,-0.345734599579915,
8.3716914957747));
#23693=CARTESIAN_POINT('Ctrl Pts',(0.329254578046856,-0.353250949684936,
8.58095279849071));
#23694=CARTESIAN_POINT('Ctrl Pts',(0.758488001187141,-0.360767299789957,
9.03515948120896));
#23695=CARTESIAN_POINT('Ctrl Pts',(0.934107096026125,-0.368283649894978,
9.63498649925687));
#23696=CARTESIAN_POINT('Ctrl Pts',(0.856422329660891,-0.373294549964993,
10.0442235818997));
#23697=CARTESIAN_POINT('Ctrl Pts',(0.773161008253379,-0.3758,10.228905014477));
#23698=CARTESIAN_POINT('Ctrl Pts',(-1.70236438819101,-0.131276297823037,
9.60284307890691));
#23699=CARTESIAN_POINT('Ctrl Pts',(-1.68706974470556,-0.133781747858044,
9.39782218300541));
#23700=CARTESIAN_POINT('Ctrl Pts',(-1.55794454395348,-0.138792647928058,
8.99529563636627));
#23701=CARTESIAN_POINT('Ctrl Pts',(-1.1105860932347,-0.14630899803308,8.54563816797476));
#23702=CARTESIAN_POINT('Ctrl Pts',(-0.50770340381119,-0.153825348138101,
8.34875817330592));
#23703=CARTESIAN_POINT('Ctrl Pts',(0.118782788653509,-0.161341698243123,
8.44766358620418));
#23704=CARTESIAN_POINT('Ctrl Pts',(0.631686746274308,-0.168858048348144,
8.82074498963809));
#23705=CARTESIAN_POINT('Ctrl Pts',(0.918738129196869,-0.176374398453165,
9.38630714441723));
#23706=CARTESIAN_POINT('Ctrl Pts',(0.917088242876597,-0.183890748558187,
10.0205460967523));
#23707=CARTESIAN_POINT('Ctrl Pts',(0.627101574915222,-0.191407098663208,
10.5846095141902));
#23708=CARTESIAN_POINT('Ctrl Pts',(0.112260657645241,-0.19892344876823,
10.9550142627446));
#23709=CARTESIAN_POINT('Ctrl Pts',(-0.514724477672702,-0.206439798873251,
11.050670155678));
#23710=CARTESIAN_POINT('Ctrl Pts',(-1.11659415908861,-0.213956148978272,
10.8506365740717));
#23711=CARTESIAN_POINT('Ctrl Pts',(-1.56158651998784,-0.221472499083294,
10.3987048019213));
#23712=CARTESIAN_POINT('Ctrl Pts',(-1.75228360744098,-0.228988849188315,
9.79381213789479));
#23713=CARTESIAN_POINT('Ctrl Pts',(-1.6469378544924,-0.236505199293337,
9.16838204421781));
#23714=CARTESIAN_POINT('Ctrl Pts',(-1.26861163914299,-0.244021549398358,
8.65933411469724));
#23715=CARTESIAN_POINT('Ctrl Pts',(-0.700128381796828,-0.25153789950338,
8.37810945216957));
#23716=CARTESIAN_POINT('Ctrl Pts',(-0.0659408198066945,-0.259054249608401,
8.38627395234078));
#23717=CARTESIAN_POINT('Ctrl Pts',(0.495114283874633,-0.266570599713422,
8.68204023419045));
#23718=CARTESIAN_POINT('Ctrl Pts',(0.860210371183234,-0.274086949818444,
9.20065894936438));
#23719=CARTESIAN_POINT('Ctrl Pts',(0.949420362504933,-0.281603299923465,
9.82859373675729));
#23720=CARTESIAN_POINT('Ctrl Pts',(0.743214348685499,-0.289119650028487,
10.42837670551));
#23721=CARTESIAN_POINT('Ctrl Pts',(0.286735084002856,-0.296636000133508,
10.8687029426013));
#23722=CARTESIAN_POINT('Ctrl Pts',(-0.320084677783521,-0.304152350238529,
11.0531759884458));
#23723=CARTESIAN_POINT('Ctrl Pts',(-0.944399567770392,-0.311668700343551,
10.9414107643435));
#23724=CARTESIAN_POINT('Ctrl Pts',(-1.44953411414706,-0.319185050448572,
10.5578752381932));
#23725=CARTESIAN_POINT('Ctrl Pts',(-1.72490401001437,-0.326701400553594,
9.98653272419914));
#23726=CARTESIAN_POINT('Ctrl Pts',(-1.7102249118596,-0.334217750658615,
9.35246306669736));
#23727=CARTESIAN_POINT('Ctrl Pts',(-1.40871077469487,-0.341734100763636,
8.79447471926191));
#23728=CARTESIAN_POINT('Ctrl Pts',(-0.886368443796752,-0.349250450868658,
8.43472822976116));
#23729=CARTESIAN_POINT('Ctrl Pts',(-0.257551350854068,-0.35676680097368,
8.35196793158375));
#23730=CARTESIAN_POINT('Ctrl Pts',(0.340083010926646,-0.364283151078701,
8.56433647838023));
#23731=CARTESIAN_POINT('Ctrl Pts',(0.775689963218691,-0.371799501183722,
9.02528750899211));
#23732=CARTESIAN_POINT('Ctrl Pts',(0.953916761372978,-0.379315851288744,
9.63402113770787));
#23733=CARTESIAN_POINT('Ctrl Pts',(0.875078482498271,-0.384326751358758,
10.0493348312006));
#23734=CARTESIAN_POINT('Ctrl Pts',(0.790580844367512,-0.386832201393765,
10.2367585304116));
#23735=CARTESIAN_POINT('Ctrl Pts',(-1.72141977137688,-0.142308499216802,
9.60142153945346));
#23736=CARTESIAN_POINT('Ctrl Pts',(-1.70590134621024,-0.144813949251809,
9.3934009057152));
#23737=CARTESIAN_POINT('Ctrl Pts',(-1.57488686608167,-0.149824849321823,
8.98498484178101));
#23738=CARTESIAN_POINT('Ctrl Pts',(-1.12098294561788,-0.157341199426845,
8.52874826585226));
#23739=CARTESIAN_POINT('Ctrl Pts',(-0.509279252819849,-0.164857549531866,
8.3289876459344));
#23740=CARTESIAN_POINT('Ctrl Pts',(0.126373294749698,-0.172373899636888,
8.42934018112733));
#23741=CARTESIAN_POINT('Ctrl Pts',(0.646781743078804,-0.179890249741909,
8.80788027889165));
#23742=CARTESIAN_POINT('Ctrl Pts',(0.93803308274559,-0.18740659984693,9.3817173862666));
#23743=CARTESIAN_POINT('Ctrl Pts',(0.93635905631804,-0.194922949951952,
10.025236127252));
#23744=CARTESIAN_POINT('Ctrl Pts',(0.64212948435307,-0.202439300056973,
10.597552568696));
#23745=CARTESIAN_POINT('Ctrl Pts',(0.119755735989659,-0.209955650161995,
10.9733768484366));
#23746=CARTESIAN_POINT('Ctrl Pts',(-0.516403054653671,-0.217472000267016,
11.0704323187159));
#23747=CARTESIAN_POINT('Ctrl Pts',(-1.12707891774294,-0.224988350372037,
10.867471970544));
#23748=CARTESIAN_POINT('Ctrl Pts',(-1.57858212923714,-0.232504700477059,
10.4089278146627));
#23749=CARTESIAN_POINT('Ctrl Pts',(-1.77206937749842,-0.24002105058208,
9.79518473856729));
#23750=CARTESIAN_POINT('Ctrl Pts',(-1.66518227121767,-0.247537400687102,
9.16060374196403));
#23751=CARTESIAN_POINT('Ctrl Pts',(-1.28132062272213,-0.255053750792123,
8.64410774073254));
#23752=CARTESIAN_POINT('Ctrl Pts',(-0.704519673029873,-0.262570100897145,
8.35876837439818));
#23753=CARTESIAN_POINT('Ctrl Pts',(-0.06105307430086,-0.270086451002166,
8.36705233244209));
#23754=CARTESIAN_POINT('Ctrl Pts',(0.508211037616542,-0.277602801107187,
8.66714608199988));
#23755=CARTESIAN_POINT('Ctrl Pts',(0.878648983092034,-0.285119151212209,
9.19335290264921));
#23756=CARTESIAN_POINT('Ctrl Pts',(0.969164239348842,-0.29263550131723,
9.83047524008419));
#23757=CARTESIAN_POINT('Ctrl Pts',(0.759941147786661,-0.300151851422252,
10.4390338590325));
#23758=CARTESIAN_POINT('Ctrl Pts',(0.296782963299545,-0.307668201527273,
10.8858026749064));
#23759=CARTESIAN_POINT('Ctrl Pts',(-0.318915406647834,-0.315184551632294,
11.0729748152654));
#23760=CARTESIAN_POINT('Ctrl Pts',(-0.952364882596371,-0.322700901737316,
10.9595743121341));
#23761=CARTESIAN_POINT('Ctrl Pts',(-1.46489024250333,-0.330217251842337,
10.5704271334521));
#23762=CARTESIAN_POINT('Ctrl Pts',(-1.74428917888433,-0.337733601947359,
9.99072509225252));
#23763=CARTESIAN_POINT('Ctrl Pts',(-1.72939530532362,-0.34524995205238,
9.34737812311678));
#23764=CARTESIAN_POINT('Ctrl Pts',(-1.42346960141787,-0.352766302157402,
8.78122563830929));
#23765=CARTESIAN_POINT('Ctrl Pts',(-0.893484683422232,-0.360282652262423,
8.41621556261918));
#23766=CARTESIAN_POINT('Ctrl Pts',(-0.255467131093149,-0.367799002367444,
8.33224436739279));
#23767=CARTESIAN_POINT('Ctrl Pts',(0.350911443806435,-0.375315352472466,
8.54772015826975));
#23768=CARTESIAN_POINT('Ctrl Pts',(0.792891925250241,-0.382831702577487,
9.01541553677525));
#23769=CARTESIAN_POINT('Ctrl Pts',(0.973726426719832,-0.390348052682509,
9.63305577615887));
#23770=CARTESIAN_POINT('Ctrl Pts',(0.893734635335651,-0.395358952752523,
10.0544460805015));
#23771=CARTESIAN_POINT('Ctrl Pts',(0.808000680481646,-0.39786440278753,
10.2446120463461));
#23772=CARTESIAN_POINT('Ctrl Pts',(-1.74047515456274,-0.153340700610567,
9.6));
#23773=CARTESIAN_POINT('Ctrl Pts',(-1.72473294771491,-0.155846150645574,
9.38897962842498));
#23774=CARTESIAN_POINT('Ctrl Pts',(-1.59182918820986,-0.160857050715588,
8.97467404719576));
#23775=CARTESIAN_POINT('Ctrl Pts',(-1.13137979800106,-0.16837340082061,
8.51185836372975));
#23776=CARTESIAN_POINT('Ctrl Pts',(-0.510855101828509,-0.175889750925631,
8.30921711856289));
#23777=CARTESIAN_POINT('Ctrl Pts',(0.133963800845887,-0.183406101030653,
8.41101677605048));
#23778=CARTESIAN_POINT('Ctrl Pts',(0.6618767398833,-0.190922451135674,8.79501556814522));
#23779=CARTESIAN_POINT('Ctrl Pts',(0.957328036294311,-0.198438801240695,
9.37712762811596));
#23780=CARTESIAN_POINT('Ctrl Pts',(0.955629869759482,-0.205955151345717,
10.0299261577517));
#23781=CARTESIAN_POINT('Ctrl Pts',(0.657157393790918,-0.213471501450738,
10.6104956232018));
#23782=CARTESIAN_POINT('Ctrl Pts',(0.127250814334077,-0.22098785155576,
10.9917394341285));
#23783=CARTESIAN_POINT('Ctrl Pts',(-0.51808163163464,-0.228504201660781,
11.0901944817538));
#23784=CARTESIAN_POINT('Ctrl Pts',(-1.13756367639728,-0.236020551765803,
10.8843073670163));
#23785=CARTESIAN_POINT('Ctrl Pts',(-1.59557773848644,-0.243536901870824,
10.4191508274041));
#23786=CARTESIAN_POINT('Ctrl Pts',(-1.79185514755587,-0.251053251975845,
9.79655733923979));
#23787=CARTESIAN_POINT('Ctrl Pts',(-1.68342668794294,-0.258569602080867,
9.15282543971024));
#23788=CARTESIAN_POINT('Ctrl Pts',(-1.29402960630127,-0.266085952185888,
8.62888136676785));
#23789=CARTESIAN_POINT('Ctrl Pts',(-0.708910964262916,-0.27360230229091,
8.3394272966268));
#23790=CARTESIAN_POINT('Ctrl Pts',(-0.0561653287950267,-0.281118652395931,
8.34783071254341));
#23791=CARTESIAN_POINT('Ctrl Pts',(0.521307791358451,-0.288635002500952,
8.65225192980931));
#23792=CARTESIAN_POINT('Ctrl Pts',(0.897087595000832,-0.296151352605974,
9.18604685593405));
#23793=CARTESIAN_POINT('Ctrl Pts',(0.988908116192752,-0.303667702710995,
9.83235674341108));
#23794=CARTESIAN_POINT('Ctrl Pts',(0.776667946887822,-0.311184052816017,
10.4496910125549));
#23795=CARTESIAN_POINT('Ctrl Pts',(0.306830842596235,-0.318700402921038,
10.9029024072114));
#23796=CARTESIAN_POINT('Ctrl Pts',(-0.317746135512149,-0.32621675302606,
11.0927736420849));
#23797=CARTESIAN_POINT('Ctrl Pts',(-0.960330197422347,-0.333733103131081,
10.9777378599246));
#23798=CARTESIAN_POINT('Ctrl Pts',(-1.48024637085961,-0.341249453236102,
10.5829790287109));
#23799=CARTESIAN_POINT('Ctrl Pts',(-1.7636743477543,-0.348765803341124,
9.99491746030589));
#23800=CARTESIAN_POINT('Ctrl Pts',(-1.74856569878764,-0.356282153446145,
9.34229317953619));
#23801=CARTESIAN_POINT('Ctrl Pts',(-1.43822842814087,-0.363798503551167,
8.76797655735667));
#23802=CARTESIAN_POINT('Ctrl Pts',(-0.900600923047711,-0.371314853656188,
8.39770289547719));
#23803=CARTESIAN_POINT('Ctrl Pts',(-0.253382911332231,-0.37883120376121,
8.31252080320183));
#23804=CARTESIAN_POINT('Ctrl Pts',(0.361739876686224,-0.386347553866231,
8.53110383815927));
#23805=CARTESIAN_POINT('Ctrl Pts',(0.810093887281791,-0.393863903971252,
9.0055435645584));
#23806=CARTESIAN_POINT('Ctrl Pts',(0.993536092066686,-0.401380254076274,
9.63209041460987));
#23807=CARTESIAN_POINT('Ctrl Pts',(0.912390788173031,-0.406391154146288,
10.0595573298025));
#23808=CARTESIAN_POINT('Ctrl Pts',(0.825420516595779,-0.408896604181295,
10.2524655622807));
#23809=CARTESIAN_POINT('',(0.938792124585917,-0.2,9.6));
#23810=CARTESIAN_POINT('',(0.882983735526293,-0.167820985845947,9.6));
#23811=CARTESIAN_POINT('Ctrl Pts',(0.938792124585917,-0.2,9.6));
#23812=CARTESIAN_POINT('Ctrl Pts',(0.92977267608958,-0.194799120566257,
9.6));
#23813=CARTESIAN_POINT('Ctrl Pts',(0.920750513898092,-0.189596807415628,
9.6));
#23814=CARTESIAN_POINT('Ctrl Pts',(0.902150020937586,-0.178871773266908,
9.6));
#23815=CARTESIAN_POINT('Ctrl Pts',(0.892565160581531,-0.17334530521579,
9.6));
#23816=CARTESIAN_POINT('Ctrl Pts',(0.882983735526293,-0.167820985845947,
9.6));
#23817=CARTESIAN_POINT('',(0.934663813609417,-0.2,9.8));
#23818=CARTESIAN_POINT('Ctrl Pts',(0.934605726336547,-0.2,9.80001655533327));
#23819=CARTESIAN_POINT('Ctrl Pts',(0.939837723241998,-0.2,9.74496032472243));
#23820=CARTESIAN_POINT('Ctrl Pts',(0.941679232433745,-0.2,9.689639007292));
#23821=CARTESIAN_POINT('Ctrl Pts',(0.940136539876103,-0.2,9.6343742241444));
#23822=CARTESIAN_POINT('Ctrl Pts',(0.939816429070574,-0.2,9.62290670641825));
#23823=CARTESIAN_POINT('Ctrl Pts',(0.939350427036596,-0.2,9.61144160667945));
#23824=CARTESIAN_POINT('Ctrl Pts',(0.938738309086801,-0.2,9.59998178926018));
#23825=CARTESIAN_POINT('',(0.882983735526293,-0.170296992535546,9.8));
#23826=CARTESIAN_POINT('Ctrl Pts',(0.882983735526293,-0.170296992535546,
9.8));
#23827=CARTESIAN_POINT('Ctrl Pts',(0.89256533649203,-0.175802996473857,
9.8));
#23828=CARTESIAN_POINT('Ctrl Pts',(0.902150185403708,-0.181311444968124,
9.8));
#23829=CARTESIAN_POINT('Ctrl Pts',(0.919374602560811,-0.191211354334495,
9.8));
#23830=CARTESIAN_POINT('Ctrl Pts',(0.927019922390104,-0.195605924238071,
9.8));
#23831=CARTESIAN_POINT('Ctrl Pts',(0.934663813609417,-0.2,9.8));
#23832=CARTESIAN_POINT('Ctrl Pts',(0.882930320251132,-0.170296992535546,
9.80001652754054));
#23833=CARTESIAN_POINT('Ctrl Pts',(0.877609657584953,-0.171150844078505,
9.86885824031965));
#23834=CARTESIAN_POINT('Ctrl Pts',(0.835029778105595,-0.17451014565647,
10.1379865677368));
#23835=CARTESIAN_POINT('Ctrl Pts',(0.612073665477375,-0.180374897269443,
10.5716664596844));
#23836=CARTESIAN_POINT('Ctrl Pts',(0.104765579300823,-0.187891247374464,
10.9366516770526));
#23837=CARTESIAN_POINT('Ctrl Pts',(-0.513045900691733,-0.195407597479486,
11.0309079926402));
#23838=CARTESIAN_POINT('Ctrl Pts',(-1.10610940043427,-0.202923947584507,
10.8338011775994));
#23839=CARTESIAN_POINT('Ctrl Pts',(-1.54459091073853,-0.210440297689529,
10.3884817891799));
#23840=CARTESIAN_POINT('Ctrl Pts',(-1.6790482842046,-0.215818644891609,
9.96198194106933));
#23841=CARTESIAN_POINT('Ctrl Pts',(-1.68694501923047,-0.218691542058681,
9.72972816411997));
#23842=CARTESIAN_POINT('Ctrl Pts',(-1.6869212373449,-0.219058989190747,
9.70002100226366));
#23843=CARTESIAN_POINT('',(-0.514332464396186,-0.3758,8.36074669039516));
#23844=CARTESIAN_POINT('Ctrl Pts',(-0.5143324643962,-0.3758,8.36074669039516));
#23845=CARTESIAN_POINT('Ctrl Pts',(-0.459186112744666,-0.3758,8.35715151017609));
#23846=CARTESIAN_POINT('Ctrl Pts',(-0.403937654194788,-0.3758,8.35693183338276));
#23847=CARTESIAN_POINT('Ctrl Pts',(-0.348901189845087,-0.3758,8.36012059653181));
#23848=CARTESIAN_POINT('Ctrl Pts',(-0.318949026847784,-0.3758,8.36185599786488));
#23849=CARTESIAN_POINT('Ctrl Pts',(-0.289059567473804,-0.3758,8.36460180455001));
#23850=CARTESIAN_POINT('Ctrl Pts',(-0.259283881757075,-0.3758,8.36836982212099));
#23851=CARTESIAN_POINT('Ctrl Pts',(-0.238690403378431,-0.3758,8.37097586079015));
#23852=CARTESIAN_POINT('Ctrl Pts',(-0.218151358285065,-0.3758,8.3740709655289));
#23853=CARTESIAN_POINT('Ctrl Pts',(-0.197682861612178,-0.3758,8.37764974829637));
#23854=CARTESIAN_POINT('Ctrl Pts',(-0.185643896254699,-0.3758,8.37975468264734));
#23855=CARTESIAN_POINT('Ctrl Pts',(-0.173627293719959,-0.3758,8.3820273824134));
#23856=CARTESIAN_POINT('Ctrl Pts',(-0.161642970436637,-0.3758,8.38446555730322));
#23857=CARTESIAN_POINT('Ctrl Pts',(-0.107637690513597,-0.3758,8.39545277070804));
#23858=CARTESIAN_POINT('Ctrl Pts',(-0.0544133015938191,-0.3758,8.40976919406099));
#23859=CARTESIAN_POINT('Ctrl Pts',(-0.00226237454520876,-0.3758,8.42727966409744));
#23860=CARTESIAN_POINT('Ctrl Pts',(0.030941959568332,-0.3758,8.43842852626499));
#23861=CARTESIAN_POINT('Ctrl Pts',(0.0637110029072512,-0.3758,8.45087327629095));
#23862=CARTESIAN_POINT('Ctrl Pts',(0.0959655247076156,-0.3758,8.46458937152845));
#23863=CARTESIAN_POINT('Ctrl Pts',(0.115792643065664,-0.3758,8.47302076745388));
#23864=CARTESIAN_POINT('Ctrl Pts',(0.135425272733956,-0.3758,8.48193271440877));
#23865=CARTESIAN_POINT('Ctrl Pts',(0.154844151472763,-0.3758,8.49132089519076));
#23866=CARTESIAN_POINT('Ctrl Pts',(0.164400066961461,-0.3758,8.49594076348243));
#23867=CARTESIAN_POINT('Ctrl Pts',(0.173903375406978,-0.3758,8.5006756813438));
#23868=CARTESIAN_POINT('Ctrl Pts',(0.18334038592269,-0.3758,8.50551899364961));
#23869=CARTESIAN_POINT('Ctrl Pts',(0.231990305124483,-0.3758,8.53048736175241));
#23870=CARTESIAN_POINT('Ctrl Pts',(0.278961911005049,-0.3758,8.55837168896474));
#23871=CARTESIAN_POINT('Ctrl Pts',(0.323970100024214,-0.3758,8.58905342668914));
#23872=CARTESIAN_POINT('Ctrl Pts',(0.369162236320362,-0.3758,8.61986055986335));
#23873=CARTESIAN_POINT('Ctrl Pts',(0.41237579564963,-0.3758,8.6534885441088));
#23874=CARTESIAN_POINT('Ctrl Pts',(0.453401593903601,-0.3758,8.68969605386198));
#23875=CARTESIAN_POINT('Ctrl Pts',(0.482061638209065,-0.3758,8.71499010974586));
#23876=CARTESIAN_POINT('Ctrl Pts',(0.509653403937738,-0.3758,8.74154398427469));
#23877=CARTESIAN_POINT('Ctrl Pts',(0.536094141849884,-0.3758,8.76928524079275));
#23878=CARTESIAN_POINT('Ctrl Pts',(0.545597327910121,-0.3758,8.77925585216947));
#23879=CARTESIAN_POINT('Ctrl Pts',(0.554951726191651,-0.3758,8.78937991159023));
#23880=CARTESIAN_POINT('Ctrl Pts',(0.564153143107668,-0.3758,8.79965425101923));
#23881=CARTESIAN_POINT('Ctrl Pts',(0.570667013019575,-0.3758,8.8069276645687));
#23882=CARTESIAN_POINT('Ctrl Pts',(0.577103878399466,-0.3758,8.814276170528));
#23883=CARTESIAN_POINT('Ctrl Pts',(0.583453562357181,-0.3758,8.82168809871078));
#23884=CARTESIAN_POINT('Ctrl Pts',(0.618945997994518,-0.3758,8.8631180951843));
#23885=CARTESIAN_POINT('Ctrl Pts',(0.651791132138043,-0.3758,8.90660779224594));
#23886=CARTESIAN_POINT('Ctrl Pts',(0.681792858457505,-0.3758,8.95191277562012));
#23887=CARTESIAN_POINT('Ctrl Pts',(0.70212728285197,-0.3758,8.98261936727772));
#23888=CARTESIAN_POINT('Ctrl Pts',(0.721154825564954,-0.3758,9.014160730134));
#23889=CARTESIAN_POINT('Ctrl Pts',(0.738803455298371,-0.3758,9.04646884572015));
#23890=CARTESIAN_POINT('Ctrl Pts',(0.763421765357715,-0.3758,9.09153586899318));
#23891=CARTESIAN_POINT('Ctrl Pts',(0.78535872190006,-0.3758,9.13809472230648));
#23892=CARTESIAN_POINT('Ctrl Pts',(0.804529778979719,-0.3758,9.18588977192258));
#23893=CARTESIAN_POINT('Ctrl Pts',(0.80997310737791,-0.3758,9.1994604451404));
#23894=CARTESIAN_POINT('Ctrl Pts',(0.815193201908606,-0.3758,9.21313083794842));
#23895=CARTESIAN_POINT('Ctrl Pts',(0.820187520955781,-0.3758,9.22689519764528));
#23896=CARTESIAN_POINT('Ctrl Pts',(0.824722129234267,-0.3758,9.2393925929538));
#23897=CARTESIAN_POINT('Ctrl Pts',(0.829071936284644,-0.3758,9.25197198301473));
#23898=CARTESIAN_POINT('Ctrl Pts',(0.833226054633313,-0.3758,9.26460086536546));
#23899=CARTESIAN_POINT('Ctrl Pts',(0.850147611958222,-0.3758,9.31604387654393));
#23900=CARTESIAN_POINT('Ctrl Pts',(0.863857203739219,-0.3758,9.36838576470231));
#23901=CARTESIAN_POINT('Ctrl Pts',(0.87429910262014,-0.3758,9.42131543047171));
#23902=CARTESIAN_POINT('Ctrl Pts',(0.884689718113437,-0.3758,9.47398514231917));
#23903=CARTESIAN_POINT('Ctrl Pts',(0.891844862197499,-0.3758,9.52723792662456));
#23904=CARTESIAN_POINT('Ctrl Pts',(0.895659916756747,-0.3758,9.58077807753031));
#23905=CARTESIAN_POINT('Ctrl Pts',(0.896985769943157,-0.3758,9.59938498827741));
#23906=CARTESIAN_POINT('Ctrl Pts',(0.897907756370869,-0.3758,9.61802662991583));
#23907=CARTESIAN_POINT('Ctrl Pts',(0.898419996116996,-0.3758,9.63669054313271));
#23908=CARTESIAN_POINT('Ctrl Pts',(0.89914203714867,-0.3758,9.66299875380179));
#23909=CARTESIAN_POINT('Ctrl Pts',(0.899050055209692,-0.3758,9.68935126075387));
#23910=CARTESIAN_POINT('Ctrl Pts',(0.898148036015986,-0.3758,9.71571189798373));
#23911=CARTESIAN_POINT('Ctrl Pts',(0.897793169615475,-0.3758,9.72608252481098));
#23912=CARTESIAN_POINT('Ctrl Pts',(0.897312803258196,-0.3758,9.73645602369309));
#23913=CARTESIAN_POINT('Ctrl Pts',(0.896707362381433,-0.3758,9.74682507694203));
#23914=CARTESIAN_POINT('Ctrl Pts',(0.893575068153731,-0.3758,9.80047015920346));
#23915=CARTESIAN_POINT('Ctrl Pts',(0.887113972407378,-0.3758,9.85376450073757));
#23916=CARTESIAN_POINT('Ctrl Pts',(0.877430475724668,-0.3758,9.90640969563552));
#23917=CARTESIAN_POINT('Ctrl Pts',(0.86771391187951,-0.3758,9.95923466311653));
#23918=CARTESIAN_POINT('Ctrl Pts',(0.854752661161743,-0.3758,10.0114071099657));
#23919=CARTESIAN_POINT('Ctrl Pts',(0.838602504381783,-0.3758,10.0626183118125));
#23920=CARTESIAN_POINT('Ctrl Pts',(0.822752772426385,-0.3758,10.112876884125));
#23921=CARTESIAN_POINT('Ctrl Pts',(0.803831305864454,-0.3758,10.1622105740949));
#23922=CARTESIAN_POINT('Ctrl Pts',(0.781845869462943,-0.3758,10.2103058753372));
#23923=CARTESIAN_POINT('Ctrl Pts',(0.77900224348841,-0.3758,10.2165265864191));
#23924=CARTESIAN_POINT('Ctrl Pts',(0.776107301341429,-0.3758,10.2227265387929));
#23925=CARTESIAN_POINT('Ctrl Pts',(0.773161008253381,-0.3758,10.228905014477));
#23926=CARTESIAN_POINT('Ctrl Pts',(-1.74411350535466,-0.352155593372042,
9.70000771515446));
#23927=CARTESIAN_POINT('Ctrl Pts',(-1.74408777242683,-0.353531113396743,
9.58381303222107));
#23928=CARTESIAN_POINT('Ctrl Pts',(-1.72913983536605,-0.354906633421444,
9.46761183026196));
#23929=CARTESIAN_POINT('Ctrl Pts',(-1.69936092850762,-0.356282153446145,
9.35534445596789));
#23930=CARTESIAN_POINT('Ctrl Pts',(-1.64511994190538,-0.358787603481153,
9.15085430547635));
#23931=CARTESIAN_POINT('Ctrl Pts',(-1.54167418502313,-0.36129305351616,
8.95941543141651));
#23932=CARTESIAN_POINT('Ctrl Pts',(-1.40034672239981,-0.363798503551167,
8.80198371740668));
#23933=CARTESIAN_POINT('Ctrl Pts',(-1.25901925977648,-0.366303953586174,
8.64455200339684));
#23934=CARTESIAN_POINT('Ctrl Pts',(-1.0798100914121,-0.368809403621181,
8.52112744943702));
#23935=CARTESIAN_POINT('Ctrl Pts',(-0.882335838610658,-0.371314853656188,
8.44521815707788));
#23936=CARTESIAN_POINT('Ctrl Pts',(-0.764499267592279,-0.372809902437459,
8.39992166605114));
#23937=CARTESIAN_POINT('Ctrl Pts',(-0.64015899031043,-0.374304951218729,
8.37154408418945));
#23938=CARTESIAN_POINT('Ctrl Pts',(-0.514332464396186,-0.3758,8.36074669039516));
#23939=CARTESIAN_POINT('',(-1.70717578408079,-0.134200000000245,9.59999999967343));
#23940=CARTESIAN_POINT('Ctrl Pts',(-1.70717578408079,-0.134200000000245,
9.59999999967343));
#23941=CARTESIAN_POINT('Ctrl Pts',(-1.70869435368597,-0.135072786034822,
9.59999999967343));
#23942=CARTESIAN_POINT('Ctrl Pts',(-1.71021285656339,-0.135945547417202,
9.6));
#23943=CARTESIAN_POINT('Ctrl Pts',(-1.72131168622386,-0.14232471291867,
9.6));
#23944=CARTESIAN_POINT('Ctrl Pts',(-1.73089522164145,-0.147833488670363,
9.6));
#23945=CARTESIAN_POINT('Ctrl Pts',(-1.74047515456274,-0.153340700610567,
9.6));
#23946=CARTESIAN_POINT('',(-1.14715243039944,-0.134200000000245,8.65223546950032));
#23947=CARTESIAN_POINT('Ctrl Pts',(-1.14715616136387,-0.134200000000245,
8.65218366173329));
#23948=CARTESIAN_POINT('Ctrl Pts',(-1.1914614130295,-0.134200000000245,
8.68241986696621));
#23949=CARTESIAN_POINT('Ctrl Pts',(-1.23378474695924,-0.134200000000245,
8.71538107777202));
#23950=CARTESIAN_POINT('Ctrl Pts',(-1.27392321752278,-0.134200000000245,
8.75081519069846));
#23951=CARTESIAN_POINT('Ctrl Pts',(-1.30598751675522,-0.134200000000245,
8.77912145110046));
#23952=CARTESIAN_POINT('Ctrl Pts',(-1.33665733147895,-0.134200000000245,
8.80900694133707));
#23953=CARTESIAN_POINT('Ctrl Pts',(-1.36581520383624,-0.134200000000245,
8.84036234914257));
#23954=CARTESIAN_POINT('Ctrl Pts',(-1.37659359337313,-0.134200000000245,
8.85195307137615));
#23955=CARTESIAN_POINT('Ctrl Pts',(-1.38716523755777,-0.134200000000245,
8.86374479838921));
#23956=CARTESIAN_POINT('Ctrl Pts',(-1.39752365245874,-0.134200000000245,
8.87573248846776));
#23957=CARTESIAN_POINT('Ctrl Pts',(-1.40511942403085,-0.134200000000245,
8.88452299902217));
#23958=CARTESIAN_POINT('Ctrl Pts',(-1.41259434273687,-0.134200000000245,
8.89341174311036));
#23959=CARTESIAN_POINT('Ctrl Pts',(-1.41994559115476,-0.134200000000245,
8.90239537788468));
#23960=CARTESIAN_POINT('Ctrl Pts',(-1.45199276022031,-0.134200000000245,
8.94155880239023));
#23961=CARTESIAN_POINT('Ctrl Pts',(-1.48169668421176,-0.134200000000245,
8.9825288838409));
#23962=CARTESIAN_POINT('Ctrl Pts',(-1.508870618509,-0.134200000000245,9.02512022251993));
#23963=CARTESIAN_POINT('Ctrl Pts',(-1.52582288453517,-0.134200000000245,
9.05169052683433));
#23964=CARTESIAN_POINT('Ctrl Pts',(-1.54178999378989,-0.134200000000245,
9.0788923978278));
#23965=CARTESIAN_POINT('Ctrl Pts',(-1.5567543716842,-0.134200000000245,
9.10666559889433));
#23966=CARTESIAN_POINT('Ctrl Pts',(-1.56527812592892,-0.134200000000245,
9.12248529699018));
#23967=CARTESIAN_POINT('Ctrl Pts',(-1.57347645003769,-0.134200000000245,
9.13849042183118));
#23968=CARTESIAN_POINT('Ctrl Pts',(-1.58134529711494,-0.134200000000245,
9.15467023201953));
#23969=CARTESIAN_POINT('Ctrl Pts',(-1.58594460208478,-0.134200000000245,
9.16412725675007));
#23970=CARTESIAN_POINT('Ctrl Pts',(-1.59042915639314,-0.134200000000245,
9.17363962921911));
#23971=CARTESIAN_POINT('Ctrl Pts',(-1.59479527804768,-0.134200000000245,
9.18319785476236));
#23972=CARTESIAN_POINT('Ctrl Pts',(-1.61725813407457,-0.134200000000245,
9.23237308652148));
#23973=CARTESIAN_POINT('Ctrl Pts',(-1.63661737531215,-0.134200000000245,
9.2828161835826));
#23974=CARTESIAN_POINT('Ctrl Pts',(-1.65281487649832,-0.134200000000245,
9.33421256568847));
#23975=CARTESIAN_POINT('Ctrl Pts',(-1.66903680873791,-0.134200000000245,
9.38568647010737));
#23976=CARTESIAN_POINT('Ctrl Pts',(-1.68208782495732,-0.134200000000244,
9.43811754687342));
#23977=CARTESIAN_POINT('Ctrl Pts',(-1.6918629726923,-0.134200000000244,
9.49121192885304));
#23978=CARTESIAN_POINT('Ctrl Pts',(-1.69848855151139,-0.134200000000244,
9.52719921233908));
#23979=CARTESIAN_POINT('Ctrl Pts',(-1.70360819823688,-0.134200000000244,
9.56349167464818));
#23980=CARTESIAN_POINT('Ctrl Pts',(-1.70717574316321,-0.134200000000244,
9.60000000632835));
#23981=CARTESIAN_POINT('Ctrl Pts',(-1.14715616136387,-0.134200000000245,
8.65218366173329));
#23982=CARTESIAN_POINT('Ctrl Pts',(-1.12354250101448,-0.134558932213268,
8.63531594196993));
#23983=CARTESIAN_POINT('Ctrl Pts',(-0.930537218441067,-0.137423314461298,
8.50712576737122));
#23984=CARTESIAN_POINT('Ctrl Pts',(-0.506127554802531,-0.142793146744336,
8.36852870067744));
#23985=CARTESIAN_POINT('Ctrl Pts',(0.111192282557321,-0.150309496849357,
8.46598699128103));
#23986=CARTESIAN_POINT('Ctrl Pts',(0.616591749469812,-0.157825846954379,
8.83360970038453));
#23987=CARTESIAN_POINT('Ctrl Pts',(0.836252869028476,-0.163663009953242,
9.26639638419685));
#23988=CARTESIAN_POINT('Ctrl Pts',(0.877788525907663,-0.166994722917098,
9.53336507663716));
#23989=CARTESIAN_POINT('Ctrl Pts',(0.882934918736163,-0.167820985845947,
9.59998192031225));
#23990=CARTESIAN_POINT('Origin',(-0.4,-0.134200000000245,9.7));
#23991=CARTESIAN_POINT('',(0.940475154562985,-0.134200000000245,9.8));
#23992=CARTESIAN_POINT('',(0.911390797333273,-0.134200000000245,9.80000000017706));
#23993=CARTESIAN_POINT('',(0.3,-0.134200000000245,9.8));
#23994=CARTESIAN_POINT('',(0.175723864053005,-0.134200000000245,10.9146668976966));
#23995=CARTESIAN_POINT('Origin',(-0.4,-0.1342,9.7));
#23996=CARTESIAN_POINT('Ctrl Pts',(0.176129947875695,-0.134200000000245,
10.9150835725709));
#23997=CARTESIAN_POINT('Ctrl Pts',(0.198206219307209,-0.134200000000245,
10.9040341608737));
#23998=CARTESIAN_POINT('Ctrl Pts',(0.219948760930549,-0.134200000000245,
10.8923781854623));
#23999=CARTESIAN_POINT('Ctrl Pts',(0.241329692205113,-0.134200000000245,
10.8801261273095));
#24000=CARTESIAN_POINT('Ctrl Pts',(0.289254661940267,-0.134200000000245,
10.852663361136));
#24001=CARTESIAN_POINT('Ctrl Pts',(0.335364934801413,-0.134200000000245,
10.8222085932717));
#24002=CARTESIAN_POINT('Ctrl Pts',(0.37946815304655,-0.134200000000245,
10.7890106425309));
#24003=CARTESIAN_POINT('Ctrl Pts',(0.408853584657123,-0.134200000000245,
10.7668912564653));
#24004=CARTESIAN_POINT('Ctrl Pts',(0.437347467573836,-0.134200000000245,
10.7435530764034));
#24005=CARTESIAN_POINT('Ctrl Pts',(0.464884284027698,-0.134200000000245,
10.7190603557891));
#24006=CARTESIAN_POINT('Ctrl Pts',(0.473497528744165,-0.134200000000245,
10.7113992742412));
#24007=CARTESIAN_POINT('Ctrl Pts',(0.482009956489796,-0.134200000000245,
10.7036315198068));
#24008=CARTESIAN_POINT('Ctrl Pts',(0.490419673663885,-0.134200000000245,
10.695759684914));
#24009=CARTESIAN_POINT('Ctrl Pts',(0.530763113022545,-0.134200000000245,
10.6579965964454));
#24010=CARTESIAN_POINT('Ctrl Pts',(0.568747696285602,-0.134200000000245,
10.6178394709025));
#24011=CARTESIAN_POINT('Ctrl Pts',(0.604171126971739,-0.134200000000245,
10.5755260135067));
#24012=CARTESIAN_POINT('Ctrl Pts',(0.626117013454232,-0.134200000000245,
10.5493115471294));
#24013=CARTESIAN_POINT('Ctrl Pts',(0.647079204216221,-0.134200000000245,
10.5222686612886));
#24014=CARTESIAN_POINT('Ctrl Pts',(0.667001543377484,-0.134200000000245,
10.4944478859121));
#24015=CARTESIAN_POINT('Ctrl Pts',(0.675322521123416,-0.134200000000245,
10.4828279626236));
#24016=CARTESIAN_POINT('Ctrl Pts',(0.6834620162914,-0.134200000000245,10.4710722913384));
#24017=CARTESIAN_POINT('Ctrl Pts',(0.691415568045136,-0.134200000000245,
10.4591843752824));
#24018=CARTESIAN_POINT('Ctrl Pts',(0.6977908946228,-0.134200000000245,10.4496553812516));
#24019=CARTESIAN_POINT('Ctrl Pts',(0.704042066980966,-0.134200000000245,
10.4400483233876));
#24020=CARTESIAN_POINT('Ctrl Pts',(0.710164383835293,-0.134200000000245,
10.4303700616719));
#24021=CARTESIAN_POINT('Ctrl Pts',(0.739480248268273,-0.134200000000245,
10.3840270488624));
#24022=CARTESIAN_POINT('Ctrl Pts',(0.765867642510717,-0.134200000000245,
10.3360201025942));
#24023=CARTESIAN_POINT('Ctrl Pts',(0.789126895014165,-0.134200000000245,
10.2865747717069));
#24024=CARTESIAN_POINT('Ctrl Pts',(0.798476858430171,-0.134200000000245,
10.2666982930961));
#24025=CARTESIAN_POINT('Ctrl Pts',(0.807320848203325,-0.134200000000245,
10.2465890474885));
#24026=CARTESIAN_POINT('Ctrl Pts',(0.815643802636578,-0.134200000000245,
10.226260533697));
#24027=CARTESIAN_POINT('Ctrl Pts',(0.836342359052429,-0.134200000000245,
10.1757050617263));
#24028=CARTESIAN_POINT('Ctrl Pts',(0.853822018600959,-0.134200000000245,
10.1237940561666));
#24029=CARTESIAN_POINT('Ctrl Pts',(0.868036229685716,-0.134200000000245,
10.0708733149591));
#24030=CARTESIAN_POINT('Ctrl Pts',(0.874996360496826,-0.134200000000245,
10.0449601440325));
#24031=CARTESIAN_POINT('Ctrl Pts',(0.881172765951885,-0.134200000000245,
10.0188047170997));
#24032=CARTESIAN_POINT('Ctrl Pts',(0.886555417284674,-0.134200000000245,
9.9924474119145));
#24033=CARTESIAN_POINT('Ctrl Pts',(0.888524749963501,-0.134200000000245,
9.98280415263246));
#24034=CARTESIAN_POINT('Ctrl Pts',(0.890387666143772,-0.134200000000245,
9.97313401876206));
#24035=CARTESIAN_POINT('Ctrl Pts',(0.892141380051336,-0.134200000000245,
9.9634529226972));
#24036=CARTESIAN_POINT('Ctrl Pts',(0.901950899807882,-0.134200000000245,
9.90930104381685));
#24037=CARTESIAN_POINT('Ctrl Pts',(0.90837109872301,-0.134200000000245,
9.85469798328913));
#24038=CARTESIAN_POINT('Ctrl Pts',(0.911390797333273,-0.134200000000245,
9.80000000035412));
#24039=CARTESIAN_POINT('Origin',(-0.4,-0.134200000000245,9.7));
#24040=CARTESIAN_POINT('',(-1.74047515456298,-0.134200000000245,9.6));
#24041=CARTESIAN_POINT('',(-1.1,-0.134200000000245,9.6));
#24042=CARTESIAN_POINT('',(0.940475154562985,-0.134200000000245,9.6));
#24043=CARTESIAN_POINT('Origin',(-0.4,-0.1342,9.7));
#24044=CARTESIAN_POINT('',(0.907175784144596,-0.134200000000245,9.6));
#24045=CARTESIAN_POINT('',(0.1,-0.134200000000245,9.6));
#24046=CARTESIAN_POINT('',(0.347152430399435,-0.134200000000245,8.65223546950032));
#24047=CARTESIAN_POINT('Ctrl Pts',(0.907175784144597,-0.134200000000245,
9.6));
#24048=CARTESIAN_POINT('Ctrl Pts',(0.90453538373471,-0.134200000000245,
9.57297027207912));
#24049=CARTESIAN_POINT('Ctrl Pts',(0.901034611734171,-0.134200000000245,
9.54600708743907));
#24050=CARTESIAN_POINT('Ctrl Pts',(0.896684152486396,-0.134200000000245,
9.51914778346216));
#24051=CARTESIAN_POINT('Ctrl Pts',(0.894686994277047,-0.134200000000245,
9.50681752672838));
#24052=CARTESIAN_POINT('Ctrl Pts',(0.892510728072362,-0.134200000000245,
9.49450917871624));
#24053=CARTESIAN_POINT('Ctrl Pts',(0.890156179963373,-0.134200000000245,
9.48222644915194));
#24054=CARTESIAN_POINT('Ctrl Pts',(0.888356131663543,-0.134200000000245,
9.47283632185529));
#24055=CARTESIAN_POINT('Ctrl Pts',(0.886452039893565,-0.134200000000245,
9.46346246266868));
#24056=CARTESIAN_POINT('Ctrl Pts',(0.884447124139638,-0.134200000000245,
9.45411839321025));
#24057=CARTESIAN_POINT('Ctrl Pts',(0.873091127340333,-0.134200000000245,
9.40119286621262));
#24058=CARTESIAN_POINT('Ctrl Pts',(0.858485365062411,-0.134200000000245,
9.34911826627378));
#24059=CARTESIAN_POINT('Ctrl Pts',(0.840774482262135,-0.134200000000245,
9.29817408776324));
#24060=CARTESIAN_POINT('Ctrl Pts',(0.823034248341469,-0.134200000000245,
9.24714548270357));
#24061=CARTESIAN_POINT('Ctrl Pts',(0.802178189415309,-0.134200000000245,
9.19725004063387));
#24062=CARTESIAN_POINT('Ctrl Pts',(0.778302217753888,-0.134200000000245,
9.14878475269468));
#24063=CARTESIAN_POINT('Ctrl Pts',(0.765046152196193,-0.134200000000245,
9.12187656888106));
#24064=CARTESIAN_POINT('Ctrl Pts',(0.750858347126933,-0.134200000000245,
9.09540960660686));
#24065=CARTESIAN_POINT('Ctrl Pts',(0.735749330922162,-0.134200000000245,
9.06943858140765));
#24066=CARTESIAN_POINT('Ctrl Pts',(0.726441613647345,-0.134200000000245,
9.05343946163604));
#24067=CARTESIAN_POINT('Ctrl Pts',(0.716784215230823,-0.134200000000245,
9.03762861234457));
#24068=CARTESIAN_POINT('Ctrl Pts',(0.706778867696372,-0.134200000000245,
9.02201952100148));
#24069=CARTESIAN_POINT('Ctrl Pts',(0.700542750909446,-0.134200000000245,
9.01229071186036));
#24070=CARTESIAN_POINT('Ctrl Pts',(0.694169554623091,-0.134200000000245,
9.00263770564262));
#24071=CARTESIAN_POINT('Ctrl Pts',(0.687672487303354,-0.134200000000245,
8.99308223011669));
#24072=CARTESIAN_POINT('Ctrl Pts',(0.657566969896279,-0.134200000000245,
8.94880493997611));
#24073=CARTESIAN_POINT('Ctrl Pts',(0.624758329671486,-0.134200000000245,
8.90654250878312));
#24074=CARTESIAN_POINT('Ctrl Pts',(0.589505146468692,-0.134200000000245,
8.86648555649876));
#24075=CARTESIAN_POINT('Ctrl Pts',(0.553825294071344,-0.134200000000245,
8.8259437950138));
#24076=CARTESIAN_POINT('Ctrl Pts',(0.51564061185778,-0.134200000000245,
8.78766039574739));
#24077=CARTESIAN_POINT('Ctrl Pts',(0.4751780594968,-0.134200000000245,8.75186738885961));
#24078=CARTESIAN_POINT('Ctrl Pts',(0.434715507135821,-0.134200000000245,
8.71607438197183));
#24079=CARTESIAN_POINT('Ctrl Pts',(0.391974258638634,-0.134200000000245,
8.68277097560167));
#24080=CARTESIAN_POINT('Ctrl Pts',(0.347152430399435,-0.134200000000245,
8.65223546950032));
#24081=CARTESIAN_POINT('Origin',(-0.4,-0.134200000000245,9.7));
#24082=CARTESIAN_POINT('Origin',(-0.4,-0.134200000000245,9.7));
#24083=CARTESIAN_POINT('',(-1.71139079735282,-0.134200000000245,9.8));
#24084=CARTESIAN_POINT('',(-1.74047515456298,-0.134200000000245,9.8));
#24085=CARTESIAN_POINT('',(-0.9,-0.134200000000245,9.8));
#24086=CARTESIAN_POINT('',(-0.975723864053004,-0.134200000000245,10.9146668976966));
#24087=CARTESIAN_POINT('Ctrl Pts',(-1.71139075641017,-0.134200000000245,
9.79999999241229));
#24088=CARTESIAN_POINT('Ctrl Pts',(-1.70840546976856,-0.134200000000245,
9.85403729104872));
#24089=CARTESIAN_POINT('Ctrl Pts',(-1.70201613810188,-0.134200000000245,
9.90781112718742));
#24090=CARTESIAN_POINT('Ctrl Pts',(-1.69235366903268,-0.134200000000245,
9.96103460131166));
#24091=CARTESIAN_POINT('Ctrl Pts',(-1.68443878317439,-0.134200000000245,
10.0046319178627));
#24092=CARTESIAN_POINT('Ctrl Pts',(-1.67432659504433,-0.134200000000245,
10.0478603021159));
#24093=CARTESIAN_POINT('Ctrl Pts',(-1.66206395378842,-0.134200000000245,
10.0905578444579));
#24094=CARTESIAN_POINT('Ctrl Pts',(-1.65801320249372,-0.134200000000245,
10.1046622385532));
#24095=CARTESIAN_POINT('Ctrl Pts',(-1.65372761924944,-0.134200000000245,
10.1187086493849));
#24096=CARTESIAN_POINT('Ctrl Pts',(-1.64920838417779,-0.134200000000245,
10.1326910333634));
#24097=CARTESIAN_POINT('Ctrl Pts',(-1.64492382198282,-0.134200000000245,
10.1459473461773));
#24098=CARTESIAN_POINT('Ctrl Pts',(-1.64042721171054,-0.134200000000245,
10.1591513010999));
#24099=CARTESIAN_POINT('Ctrl Pts',(-1.63573065417228,-0.134200000000245,
10.1722675160761));
#24100=CARTESIAN_POINT('Ctrl Pts',(-1.61716981388927,-0.134200000000245,
10.2241029230326));
#24101=CARTESIAN_POINT('Ctrl Pts',(-1.59546815140804,-0.134200000000245,
10.2746456376427));
#24102=CARTESIAN_POINT('Ctrl Pts',(-1.57076076646457,-0.134200000000245,
10.3236030074615));
#24103=CARTESIAN_POINT('Ctrl Pts',(-1.54842667430624,-0.134200000000245,
10.3678577277349));
#24104=CARTESIAN_POINT('Ctrl Pts',(-1.52363570557235,-0.134200000000245,
10.4108175770067));
#24105=CARTESIAN_POINT('Ctrl Pts',(-1.49645283004384,-0.134200000000245,
10.4522549727563));
#24106=CARTESIAN_POINT('Ctrl Pts',(-1.4664160175259,-0.134200000000245,
10.4980428911851));
#24107=CARTESIAN_POINT('Ctrl Pts',(-1.43345876263302,-0.134200000000245,
10.5419730627871));
#24108=CARTESIAN_POINT('Ctrl Pts',(-1.39780718339101,-0.134200000000245,
10.5838327068653));
#24109=CARTESIAN_POINT('Ctrl Pts',(-1.3893242475541,-0.134200000000245,
10.5937927894878));
#24110=CARTESIAN_POINT('Ctrl Pts',(-1.38068569252885,-0.134200000000245,
10.6036384832782));
#24111=CARTESIAN_POINT('Ctrl Pts',(-1.37191344138273,-0.134200000000245,
10.6133460664041));
#24112=CARTESIAN_POINT('Ctrl Pts',(-1.33495351450469,-0.134200000000245,
10.6542468063073));
#24113=CARTESIAN_POINT('Ctrl Pts',(-1.29556659195931,-0.134200000000245,
10.6927686437194));
#24114=CARTESIAN_POINT('Ctrl Pts',(-1.25402535771013,-0.134200000000245,
10.7287345588468));
#24115=CARTESIAN_POINT('Ctrl Pts',(-1.21177760165103,-0.134200000000245,
10.7653121723003));
#24116=CARTESIAN_POINT('Ctrl Pts',(-1.16730090284931,-0.134200000000245,
10.7992470464879));
#24117=CARTESIAN_POINT('Ctrl Pts',(-1.12084074134493,-0.134200000000245,
10.8303173024355));
#24118=CARTESIAN_POINT('Ctrl Pts',(-1.07438057984054,-0.134200000000245,
10.8613875583832));
#24119=CARTESIAN_POINT('Ctrl Pts',(-1.0259361067866,-0.134200000000245,
10.889594012123));
#24120=CARTESIAN_POINT('Ctrl Pts',(-0.975723864053004,-0.134200000000245,
10.9146668976966));
#24121=CARTESIAN_POINT('Origin',(-0.4,-0.1342,9.7));
#24122=CARTESIAN_POINT('Ctrl Pts',(-1.74304790533427,-0.166903395818705,
9.64435861273087));
#24123=CARTESIAN_POINT('Ctrl Pts',(-1.73435369961947,-0.169390260154196,
9.43450160975334));
#24124=CARTESIAN_POINT('Ctrl Pts',(-1.61686806594084,-0.17436398882518,
9.01909689256477));
#24125=CARTESIAN_POINT('Ctrl Pts',(-1.17795239257679,-0.181824581831654,
8.54274435715143));
#24126=CARTESIAN_POINT('Ctrl Pts',(-0.571227429489255,-0.189285174838129,
8.31612744124815));
#24127=CARTESIAN_POINT('Ctrl Pts',(0.0724614243232401,-0.196745767844604,
8.38804338598779));
#24128=CARTESIAN_POINT('Ctrl Pts',(0.6142113106438,-0.204206360851079,8.74302009654901));
#24129=CARTESIAN_POINT('Ctrl Pts',(0.93715526549064,-0.211666953857554,
9.30445338949781));
#24130=CARTESIAN_POINT('Ctrl Pts',(0.97161381549785,-0.219127546864028,
9.95122650445237));
#24131=CARTESIAN_POINT('Ctrl Pts',(0.710155473394963,-0.226588139870503,
10.5437975996746));
#24132=CARTESIAN_POINT('Ctrl Pts',(0.209187076810929,-0.234048732876978,
10.9543248434144));
#24133=CARTESIAN_POINT('Ctrl Pts',(-0.423209735858731,-0.241509325883453,
11.0942384369162));
#24134=CARTESIAN_POINT('Ctrl Pts',(-1.05059926803272,-0.248969918889928,
10.9333532476513));
#24135=CARTESIAN_POINT('Ctrl Pts',(-1.53762571409255,-0.256430511896403,
10.5063791358829));
#24136=CARTESIAN_POINT('Ctrl Pts',(-1.77921598078853,-0.263891104902878,
9.90543339520114));
#24137=CARTESIAN_POINT('Ctrl Pts',(-1.72324833240949,-0.271351697909352,
9.26016657257637));
#24138=CARTESIAN_POINT('Ctrl Pts',(-1.38179747864361,-0.278812290915827,
8.70979127833806));
#24139=CARTESIAN_POINT('Ctrl Pts',(-0.828529470919906,-0.286272883922302,
8.373047827273));
#24140=CARTESIAN_POINT('Ctrl Pts',(-0.18280869586118,-0.293733476928777,
8.32258663486116));
#24141=CARTESIAN_POINT('Ctrl Pts',(0.416054301607959,-0.301194069935252,
8.56929451772788));
#24142=CARTESIAN_POINT('Ctrl Pts',(0.838858292162744,-0.308654662941726,
9.05994544037276));
#24143=CARTESIAN_POINT('Ctrl Pts',(0.994385717937961,-0.316115255948201,
9.68868479182157));
#24144=CARTESIAN_POINT('Ctrl Pts',(0.849082503222856,-0.323575848954676,
10.3198645945257));
#24145=CARTESIAN_POINT('Ctrl Pts',(0.434296837286034,-0.331036441961151,
10.8173137931681));
#24146=CARTESIAN_POINT('Ctrl Pts',(-0.160483306787659,-0.338497034967626,
11.0737055259114));
#24147=CARTESIAN_POINT('Ctrl Pts',(-0.806938123001907,-0.345957627974101,
11.0337358503735));
#24148=CARTESIAN_POINT('Ctrl Pts',(-1.36559670937883,-0.353418220980575,
10.7060045160499));
#24149=CARTESIAN_POINT('Ctrl Pts',(-1.71593306059597,-0.36087881398705,
10.1612707751975));
#24150=CARTESIAN_POINT('Ctrl Pts',(-1.78234948954774,-0.368339406993525,
9.51695131694362));
#24151=CARTESIAN_POINT('Ctrl Pts',(-1.62778015905473,-0.373313135664508,
9.1138728193103));
#24152=CARTESIAN_POINT('Ctrl Pts',(-1.50911575994275,-0.3758,8.94056871868047));
#24153=CARTESIAN_POINT('Ctrl Pts',(-1.72395594948115,-0.17793559721247,
9.64514957700335));
#24154=CARTESIAN_POINT('Ctrl Pts',(-1.71538533533075,-0.180422461547961,
9.43827577411898));
#24155=CARTESIAN_POINT('Ctrl Pts',(-1.59956980628701,-0.185396190218945,
9.02877619887675));
#24156=CARTESIAN_POINT('Ctrl Pts',(-1.16689349238722,-0.192856783225419,
8.55919520269185));
#24157=CARTESIAN_POINT('Ctrl Pts',(-0.56879336402393,-0.200317376231894,
8.33579973565633));
#24158=CARTESIAN_POINT('Ctrl Pts',(0.0657451987741329,-0.207777969238369,
8.40669336686818));
#24159=CARTESIAN_POINT('Ctrl Pts',(0.599793896721602,-0.215238562244844,
8.7566239434382));
#24160=CARTESIAN_POINT('Ctrl Pts',(0.918147075837748,-0.222699155251319,
9.31007624062289));
#24161=CARTESIAN_POINT('Ctrl Pts',(0.952115783961518,-0.230159748257794,
9.94765522057405));
#24162=CARTESIAN_POINT('Ctrl Pts',(0.694374175345971,-0.237620341264268,
10.531802683888));
#24163=CARTESIAN_POINT('Ctrl Pts',(0.200527242168716,-0.245080934270743,
10.9364941208908));
#24164=CARTESIAN_POINT('Ctrl Pts',(-0.422879800306456,-0.252541527277218,
11.0744187874602));
#24165=CARTESIAN_POINT('Ctrl Pts',(-1.04135074275375,-0.260002120283693,
10.9158206446354));
#24166=CARTESIAN_POINT('Ctrl Pts',(-1.52145391573408,-0.267462713290168,
10.4949161383219));
#24167=CARTESIAN_POINT('Ctrl Pts',(-1.75960988147327,-0.274923306296642,
9.90251307843778));
#24168=CARTESIAN_POINT('Ctrl Pts',(-1.70443783529711,-0.282383899303117,
9.26641897827667));
#24169=CARTESIAN_POINT('Ctrl Pts',(-1.36784084013167,-0.289844492309592,
8.72386748598803));
#24170=CARTESIAN_POINT('Ctrl Pts',(-0.8224377554211,-0.297305085316067,
8.39191097593678));
#24171=CARTESIAN_POINT('Ctrl Pts',(-0.185896155938985,-0.304765678322542,
8.34216710928376));
#24172=CARTESIAN_POINT('Ctrl Pts',(0.404453767748991,-0.312226271329017,
8.58536794226076));
#24173=CARTESIAN_POINT('Ctrl Pts',(0.821247432767259,-0.319686864335491,
9.06904406846149));
#24174=CARTESIAN_POINT('Ctrl Pts',(0.97456397482414,-0.327147457341966,
9.68884564197007));
#24175=CARTESIAN_POINT('Ctrl Pts',(0.831326302633348,-0.334608050348441,
10.3110529747565));
#24176=CARTESIAN_POINT('Ctrl Pts',(0.422436978585092,-0.342068643354916,
10.8014307367793));
#24177=CARTESIAN_POINT('Ctrl Pts',(-0.163888131079282,-0.349529236361391,
11.0541777598863));
#24178=CARTESIAN_POINT('Ctrl Pts',(-0.801153337032289,-0.356989829367866,
11.0147762690556));
#24179=CARTESIAN_POINT('Ctrl Pts',(-1.35187037119375,-0.36445042237434,
10.6917037649507));
#24180=CARTESIAN_POINT('Ctrl Pts',(-1.69722655295854,-0.371911015380815,
10.1547136291408));
#24181=CARTESIAN_POINT('Ctrl Pts',(-1.76269884616919,-0.37937160838729,
9.51955342619229));
#24182=CARTESIAN_POINT('Ctrl Pts',(-1.61032677969209,-0.384345337058273,
9.12220484843122));
#24183=CARTESIAN_POINT('Ctrl Pts',(-1.49334924183068,-0.386832201393765,
8.9513643339663));
#24184=CARTESIAN_POINT('Ctrl Pts',(-1.70486399362803,-0.188967798606235,
9.64594054127583));
#24185=CARTESIAN_POINT('Ctrl Pts',(-1.69641697104203,-0.191454662941727,
9.44204993848462));
#24186=CARTESIAN_POINT('Ctrl Pts',(-1.58227154663317,-0.19642839161271,
9.03845550518874));
#24187=CARTESIAN_POINT('Ctrl Pts',(-1.15583459219765,-0.203888984619185,
8.57564604823227));
#24188=CARTESIAN_POINT('Ctrl Pts',(-0.566359298558604,-0.211349577625659,
8.35547203006451));
#24189=CARTESIAN_POINT('Ctrl Pts',(0.0590289732250258,-0.218810170632134,
8.42534334774857));
#24190=CARTESIAN_POINT('Ctrl Pts',(0.585376482799404,-0.226270763638609,
8.77022779032738));
#24191=CARTESIAN_POINT('Ctrl Pts',(0.899138886184857,-0.233731356645084,
9.31569909174798));
#24192=CARTESIAN_POINT('Ctrl Pts',(0.932617752425185,-0.241191949651559,
9.94408393669573));
#24193=CARTESIAN_POINT('Ctrl Pts',(0.678592877296979,-0.248652542658033,
10.5198077681013));
#24194=CARTESIAN_POINT('Ctrl Pts',(0.191867407526504,-0.256113135664508,
10.9186633983672));
#24195=CARTESIAN_POINT('Ctrl Pts',(-0.422549864754182,-0.263573728670983,
11.0545991380042));
#24196=CARTESIAN_POINT('Ctrl Pts',(-1.03210221747478,-0.271034321677458,
10.8982880416196));
#24197=CARTESIAN_POINT('Ctrl Pts',(-1.50528211737561,-0.278494914683933,
10.4834531407609));
#24198=CARTESIAN_POINT('Ctrl Pts',(-1.74000378215801,-0.285955507690408,
9.89959276167443));
#24199=CARTESIAN_POINT('Ctrl Pts',(-1.68562733818473,-0.293416100696883,
9.27267138397698));
#24200=CARTESIAN_POINT('Ctrl Pts',(-1.35388420161973,-0.300876693703357,
8.73794369363799));
#24201=CARTESIAN_POINT('Ctrl Pts',(-0.816346039922294,-0.308337286709832,
8.41077412460057));
#24202=CARTESIAN_POINT('Ctrl Pts',(-0.188983616016791,-0.315797879716307,
8.36174758370636));
#24203=CARTESIAN_POINT('Ctrl Pts',(0.392853233890022,-0.323258472722782,
8.60144136679362));
#24204=CARTESIAN_POINT('Ctrl Pts',(0.803636573371775,-0.330719065729256,
9.07814269655022));
#24205=CARTESIAN_POINT('Ctrl Pts',(0.95474223171032,-0.338179658735732,
9.68900649211857));
#24206=CARTESIAN_POINT('Ctrl Pts',(0.81357010204384,-0.345640251742206,
10.3022413549873));
#24207=CARTESIAN_POINT('Ctrl Pts',(0.410577119884148,-0.353100844748681,
10.7855476803905));
#24208=CARTESIAN_POINT('Ctrl Pts',(-0.167292955370904,-0.360561437755156,
11.0346499938612));
#24209=CARTESIAN_POINT('Ctrl Pts',(-0.79536855106267,-0.368022030761631,
10.9958166877377));
#24210=CARTESIAN_POINT('Ctrl Pts',(-1.33814403300867,-0.375482623768106,
10.6774030138515));
#24211=CARTESIAN_POINT('Ctrl Pts',(-1.67852004532112,-0.38294321677458,
10.1481564830842));
#24212=CARTESIAN_POINT('Ctrl Pts',(-1.74304820279064,-0.390403809781055,
9.52215553544096));
#24213=CARTESIAN_POINT('Ctrl Pts',(-1.59287340032944,-0.395377538452038,
9.13053687755215));
#24214=CARTESIAN_POINT('Ctrl Pts',(-1.47758272371861,-0.39786440278753,
8.96215994925213));
#24215=CARTESIAN_POINT('Ctrl Pts',(-1.68577203777491,-0.2,9.64673150554831));
#24216=CARTESIAN_POINT('Ctrl Pts',(-1.67744860675331,-0.202486864335492,
9.44582410285027));
#24217=CARTESIAN_POINT('Ctrl Pts',(-1.56497328697934,-0.207460593006475,
9.04813481150073));
#24218=CARTESIAN_POINT('Ctrl Pts',(-1.14477569200808,-0.21492118601295,
8.59209689377269));
#24219=CARTESIAN_POINT('Ctrl Pts',(-0.563925233093278,-0.222381779019424,
8.3751443244727));
#24220=CARTESIAN_POINT('Ctrl Pts',(0.0523127476759186,-0.229842372025899,
8.44399332862896));
#24221=CARTESIAN_POINT('Ctrl Pts',(0.570959068877206,-0.237302965032374,
8.78383163721656));
#24222=CARTESIAN_POINT('Ctrl Pts',(0.880130696531965,-0.244763558038849,
9.32132194287307));
#24223=CARTESIAN_POINT('Ctrl Pts',(0.913119720888853,-0.252224151045324,
9.94051265281741));
#24224=CARTESIAN_POINT('Ctrl Pts',(0.662811579247987,-0.259684744051799,
10.5078128523146));
#24225=CARTESIAN_POINT('Ctrl Pts',(0.183207572884291,-0.267145337058273,
10.9008326758436));
#24226=CARTESIAN_POINT('Ctrl Pts',(-0.422219929201908,-0.274605930064748,
11.0347794885482));
#24227=CARTESIAN_POINT('Ctrl Pts',(-1.02285369219581,-0.282066523071223,
10.8807554386038));
#24228=CARTESIAN_POINT('Ctrl Pts',(-1.48911031901715,-0.289527116077698,
10.4719901431999));
#24229=CARTESIAN_POINT('Ctrl Pts',(-1.72039768284276,-0.296987709084173,
9.89667244491107));
#24230=CARTESIAN_POINT('Ctrl Pts',(-1.66681684107236,-0.304448302090648,
9.27892378967729));
#24231=CARTESIAN_POINT('Ctrl Pts',(-1.33992756310779,-0.311908895097122,
8.75201990128797));
#24232=CARTESIAN_POINT('Ctrl Pts',(-0.810254324423489,-0.319369488103597,
8.42963727326435));
#24233=CARTESIAN_POINT('Ctrl Pts',(-0.192071076094596,-0.326830081110072,
8.38132805812896));
#24234=CARTESIAN_POINT('Ctrl Pts',(0.381252700031053,-0.334290674116547,
8.61751479132649));
#24235=CARTESIAN_POINT('Ctrl Pts',(0.786025713976292,-0.341751267123022,
9.08724132463895));
#24236=CARTESIAN_POINT('Ctrl Pts',(0.934920488596498,-0.349211860129497,
9.68916734226706));
#24237=CARTESIAN_POINT('Ctrl Pts',(0.795813901454333,-0.356672453135971,
10.2934297352181));
#24238=CARTESIAN_POINT('Ctrl Pts',(0.398717261183206,-0.364133046142446,
10.7696646240018));
#24239=CARTESIAN_POINT('Ctrl Pts',(-0.170697779662527,-0.371593639148921,
11.0151222278361));
#24240=CARTESIAN_POINT('Ctrl Pts',(-0.789583765093051,-0.379054232155396,
10.9768571064198));
#24241=CARTESIAN_POINT('Ctrl Pts',(-1.3244176948236,-0.386514825161871,
10.6631022627523));
#24242=CARTESIAN_POINT('Ctrl Pts',(-1.6598135376837,-0.393975418168346,
10.1415993370275));
#24243=CARTESIAN_POINT('Ctrl Pts',(-1.7233975594121,-0.40143601117482,9.52475764468964));
#24244=CARTESIAN_POINT('Ctrl Pts',(-1.57542002096679,-0.406409739845804,
9.13886890667307));
#24245=CARTESIAN_POINT('Ctrl Pts',(-1.46181620560655,-0.408896604181295,
8.97295556453796));
#24246=CARTESIAN_POINT('',(-1.6839879813829,-0.2,9.6));
#24247=CARTESIAN_POINT('Ctrl Pts',(-1.74047515456274,-0.167429513866972,
9.6));
#24248=CARTESIAN_POINT('Ctrl Pts',(-1.73089506684943,-0.172953691659501,
9.6));
#24249=CARTESIAN_POINT('Ctrl Pts',(-1.72131152231067,-0.178479715438561,
9.6));
#24250=CARTESIAN_POINT('Ctrl Pts',(-1.70248475920816,-0.189335216828392,
9.6));
#24251=CARTESIAN_POINT('Ctrl Pts',(-1.69323488525986,-0.194668542692852,
9.6));
#24252=CARTESIAN_POINT('Ctrl Pts',(-1.6839879813829,-0.2,9.6));
#24253=CARTESIAN_POINT('',(-1.50911575994275,-0.3758,8.94056871868047));
#24254=CARTESIAN_POINT('Ctrl Pts',(-1.50911575994275,-0.3758,8.94056871868047));
#24255=CARTESIAN_POINT('Ctrl Pts',(-1.62778015905473,-0.373313135664508,
9.1138728193103));
#24256=CARTESIAN_POINT('Ctrl Pts',(-1.70506482430123,-0.370826271329017,
9.31541206812696));
#24257=CARTESIAN_POINT('Ctrl Pts',(-1.73263775209919,-0.368339406993525,
9.52356826891094));
#24258=CARTESIAN_POINT('Ctrl Pts',(-1.74038047358967,-0.367641073538499,
9.58202036732419));
#24259=CARTESIAN_POINT('Ctrl Pts',(-1.74420324577494,-0.366942740083473,
9.64099423620048));
#24260=CARTESIAN_POINT('Ctrl Pts',(-1.74415902867232,-0.366244406628447,
9.69997584025059));
#24261=CARTESIAN_POINT('Ctrl Pts',(-0.517805766168013,-0.3758,10.9813944679847));
#24262=CARTESIAN_POINT('Ctrl Pts',(-0.571473798863773,-0.3758,10.977632916352));
#24263=CARTESIAN_POINT('Ctrl Pts',(-0.624797035828109,-0.3758,10.9705481800708));
#24264=CARTESIAN_POINT('Ctrl Pts',(-0.677458301761716,-0.3758,10.9601736550514));
#24265=CARTESIAN_POINT('Ctrl Pts',(-0.711008440479028,-0.3758,10.9535641148636));
#24266=CARTESIAN_POINT('Ctrl Pts',(-0.744290045716627,-0.3758,10.9456182389887));
#24267=CARTESIAN_POINT('Ctrl Pts',(-0.777220103052431,-0.3758,10.9363336630147));
#24268=CARTESIAN_POINT('Ctrl Pts',(-0.799475508486024,-0.3758,10.9300587877397));
#24269=CARTESIAN_POINT('Ctrl Pts',(-0.821570315753372,-0.3758,10.9231722657496));
#24270=CARTESIAN_POINT('Ctrl Pts',(-0.843482780797905,-0.3758,10.9156861543558));
#24271=CARTESIAN_POINT('Ctrl Pts',(-0.855588446079938,-0.3758,10.9115504097642));
#24272=CARTESIAN_POINT('Ctrl Pts',(-0.867631229210224,-0.3758,10.9072340293321));
#24273=CARTESIAN_POINT('Ctrl Pts',(-0.87960107211078,-0.3758,10.9027421420255));
#24274=CARTESIAN_POINT('Ctrl Pts',(-0.930072327745337,-0.3758,10.8838019441952));
#24275=CARTESIAN_POINT('Ctrl Pts',(-0.979284885390671,-0.3758,10.8617328387111));
#24276=CARTESIAN_POINT('Ctrl Pts',(-1.02697484201776,-0.3758,10.8367178463095));
#24277=CARTESIAN_POINT('Ctrl Pts',(-1.05204499272848,-0.3758,10.8235677058211));
#24278=CARTESIAN_POINT('Ctrl Pts',(-1.07669414949484,-0.3758,10.8096026090408));
#24279=CARTESIAN_POINT('Ctrl Pts',(-1.10088170510615,-0.3758,10.794843848367));
#24280=CARTESIAN_POINT('Ctrl Pts',(-1.11352407473803,-0.3758,10.7871297283152));
#24281=CARTESIAN_POINT('Ctrl Pts',(-1.12604030512265,-0.3758,10.7791987260189));
#24282=CARTESIAN_POINT('Ctrl Pts',(-1.13842435602362,-0.3758,10.7710535225835));
#24283=CARTESIAN_POINT('Ctrl Pts',(-1.1482030472703,-0.3758,10.7646219090369));
#24284=CARTESIAN_POINT('Ctrl Pts',(-1.15790039230216,-0.3758,10.7580558360237));
#24285=CARTESIAN_POINT('Ctrl Pts',(-1.16749853219555,-0.3758,10.7513672969233));
#24286=CARTESIAN_POINT('Ctrl Pts',(-1.2120559830556,-0.3758,10.7203170876537));
#24287=CARTESIAN_POINT('Ctrl Pts',(-1.25455184393653,-0.3758,10.6865836476055));
#24288=CARTESIAN_POINT('Ctrl Pts',(-1.29472316146515,-0.3758,10.6503463122791));
#24289=CARTESIAN_POINT('Ctrl Pts',(-1.29783952021344,-0.3758,10.6475351389369));
#24290=CARTESIAN_POINT('Ctrl Pts',(-1.30094187788386,-0.3758,10.6447088735864));
#24291=CARTESIAN_POINT('Ctrl Pts',(-1.30403010538241,-0.3758,10.6418675885036));
#24292=CARTESIAN_POINT('Ctrl Pts',(-1.34319865735068,-0.3758,10.6058310521814));
#24293=CARTESIAN_POINT('Ctrl Pts',(-1.3800969660312,-0.3758,10.5673814429018));
#24294=CARTESIAN_POINT('Ctrl Pts',(-1.41457339153483,-0.3758,10.5267797716794));
#24295=CARTESIAN_POINT('Ctrl Pts',(-1.43911105221392,-0.3758,10.4978826335072));
#24296=CARTESIAN_POINT('Ctrl Pts',(-1.46242130487303,-0.3758,10.4678944751422));
#24297=CARTESIAN_POINT('Ctrl Pts',(-1.48443773672276,-0.3758,10.436899968734));
#24298=CARTESIAN_POINT('Ctrl Pts',(-1.49127119047245,-0.3758,10.4272799027996));
#24299=CARTESIAN_POINT('Ctrl Pts',(-1.4979799245099,-0.3758,10.417562843613));
#24300=CARTESIAN_POINT('Ctrl Pts',(-1.50456173213983,-0.3758,10.4077512091659));
#24301=CARTESIAN_POINT('Ctrl Pts',(-1.5106180016241,-0.3758,10.3987230051172));
#24302=CARTESIAN_POINT('Ctrl Pts',(-1.51656214228904,-0.3758,10.3896215694345));
#24303=CARTESIAN_POINT('Ctrl Pts',(-1.52238919234587,-0.3758,10.3804551888474));
#24304=CARTESIAN_POINT('Ctrl Pts',(-1.55171967266354,-0.3758,10.3343161746342));
#24305=CARTESIAN_POINT('Ctrl Pts',(-1.57811814740431,-0.3758,10.2864877234515));
#24306=CARTESIAN_POINT('Ctrl Pts',(-1.60143419434819,-0.3758,10.2372537515648));
#24307=CARTESIAN_POINT('Ctrl Pts',(-1.61710964099662,-0.3758,10.2041536080688));
#24308=CARTESIAN_POINT('Ctrl Pts',(-1.63139113760222,-0.3758,10.1704173283456));
#24309=CARTESIAN_POINT('Ctrl Pts',(-1.64422209280247,-0.3758,10.1361236501866));
#24310=CARTESIAN_POINT('Ctrl Pts',(-1.66233225904678,-0.3758,10.0877200665955));
#24311=CARTESIAN_POINT('Ctrl Pts',(-1.67755451722892,-0.3758,10.038206150238));
#24312=CARTESIAN_POINT('Ctrl Pts',(-1.68985348202901,-0.3758,9.98784757926546));
#24313=CARTESIAN_POINT('Ctrl Pts',(-1.69317156065143,-0.3758,9.97426158235309));
#24314=CARTESIAN_POINT('Ctrl Pts',(-1.69627663659562,-0.3758,9.96061406017673));
#24315=CARTESIAN_POINT('Ctrl Pts',(-1.69916749124626,-0.3758,9.94691015785263));
#24316=CARTESIAN_POINT('Ctrl Pts',(-1.70127082332291,-0.3758,9.93693945340117));
#24317=CARTESIAN_POINT('Ctrl Pts',(-1.70326097513578,-0.3758,9.9269372019356));
#24318=CARTESIAN_POINT('Ctrl Pts',(-1.70513458302098,-0.3758,9.91692190030026));
#24319=CARTESIAN_POINT('Ctrl Pts',(-1.71520308234393,-0.3758,9.86310110965825));
#24320=CARTESIAN_POINT('Ctrl Pts',(-1.72193246689098,-0.3758,9.80880465306829));
#24321=CARTESIAN_POINT('Ctrl Pts',(-1.72532846690209,-0.3758,9.75435546665585));
#24322=CARTESIAN_POINT('Ctrl Pts',(-1.72873261248714,-0.3758,9.69977567957408));
#24323=CARTESIAN_POINT('Ctrl Pts',(-1.72878752413501,-0.3758,9.64504135850294));
#24324=CARTESIAN_POINT('Ctrl Pts',(-1.72544849409975,-0.3758,9.59046698644781));
#24325=CARTESIAN_POINT('Ctrl Pts',(-1.72411676342687,-0.3758,9.5687006757372));
#24326=CARTESIAN_POINT('Ctrl Pts',(-1.7222445784162,-0.3758,9.54695977687243));
#24327=CARTESIAN_POINT('Ctrl Pts',(-1.71982677669824,-0.3758,9.52526435065811));
#24328=CARTESIAN_POINT('Ctrl Pts',(-1.71674242348629,-0.3758,9.49758782241691));
#24329=CARTESIAN_POINT('Ctrl Pts',(-1.7127702432767,-0.3758,9.46998524578407));
#24330=CARTESIAN_POINT('Ctrl Pts',(-1.70792192303047,-0.3758,9.44249519427747));
#24331=CARTESIAN_POINT('Ctrl Pts',(-1.70542336310974,-0.3758,9.42832832050983));
#24332=CARTESIAN_POINT('Ctrl Pts',(-1.70269065454176,-0.3758,9.41418548078457));
#24333=CARTESIAN_POINT('Ctrl Pts',(-1.69973255612478,-0.3758,9.4001052573882));
#24334=CARTESIAN_POINT('Ctrl Pts',(-1.68842261816779,-0.3758,9.3462711955736));
#24335=CARTESIAN_POINT('Ctrl Pts',(-1.67381149882828,-0.3758,9.29327608491672));
#24336=CARTESIAN_POINT('Ctrl Pts',(-1.65605749550781,-0.3758,9.24140245052763));
#24337=CARTESIAN_POINT('Ctrl Pts',(-1.63795749962153,-0.3758,9.1885178953036));
#24338=CARTESIAN_POINT('Ctrl Pts',(-1.61659072299859,-0.3758,9.13679785435062));
#24339=CARTESIAN_POINT('Ctrl Pts',(-1.5920708746144,-0.3758,9.08655183398384));
#24340=CARTESIAN_POINT('Ctrl Pts',(-1.56755102623021,-0.3758,9.03630581361707));
#24341=CARTESIAN_POINT('Ctrl Pts',(-1.53987774784311,-0.3758,8.98753269584568));
#24342=CARTESIAN_POINT('Ctrl Pts',(-1.50911575994275,-0.3758,8.94056871868047));
#24343=CARTESIAN_POINT('Ctrl Pts',(-1.6839753812096,-0.2,9.60000168607488));
#24344=CARTESIAN_POINT('Ctrl Pts',(-1.6848605948529,-0.2,9.61556437837414));
#24345=CARTESIAN_POINT('Ctrl Pts',(-1.68546042900379,-0.2,9.63114344455712));
#24346=CARTESIAN_POINT('Ctrl Pts',(-1.68577203777491,-0.2,9.64673150554831));
#24347=CARTESIAN_POINT('Ctrl Pts',(0.940308825950845,-0.117455697191997,
9.80220514213222));
#24348=CARTESIAN_POINT('Ctrl Pts',(0.928986682109438,-0.119218793569698,
9.95068269426644));
#24349=CARTESIAN_POINT('Ctrl Pts',(0.821349148298486,-0.1245080827028,10.3914498221302));
#24350=CARTESIAN_POINT('Ctrl Pts',(0.39736170109172,-0.131560468213604,
10.8545453758264));
#24351=CARTESIAN_POINT('Ctrl Pts',(-0.317535341911524,-0.140375950102109,
11.1001939757858));
#24352=CARTESIAN_POINT('Ctrl Pts',(-1.0932013213438,-0.149191431990614,
10.9720179261902));
#24353=CARTESIAN_POINT('Ctrl Pts',(-1.62266150701246,-0.158006913879118,
10.3886265975781));
#24354=CARTESIAN_POINT('Ctrl Pts',(-1.72939729330723,-0.163296203012221,
9.94849597778708));
#24355=CARTESIAN_POINT('Ctrl Pts',(-1.74047515456274,-0.165059299389922,
9.8));
#24356=CARTESIAN_POINT('Ctrl Pts',(0.921255807191823,-0.128487898585762,
9.80075225571335));
#24357=CARTESIAN_POINT('Ctrl Pts',(0.910094612092099,-0.130250994963463,
9.94711914086446));
#24358=CARTESIAN_POINT('Ctrl Pts',(0.803987188290995,-0.135540284096565,
10.3816205901078));
#24359=CARTESIAN_POINT('Ctrl Pts',(0.386026889923967,-0.142592669607369,
10.838133057801));
#24360=CARTESIAN_POINT('Ctrl Pts',(-0.318707609561407,-0.151408151495874,
11.0802896659951));
#24361=CARTESIAN_POINT('Ctrl Pts',(-1.08334719106904,-0.160223633384379,
10.9539356895144));
#24362=CARTESIAN_POINT('Ctrl Pts',(-1.60528089130808,-0.169039115272883,
10.3788374988066));
#24363=CARTESIAN_POINT('Ctrl Pts',(-1.71049938628971,-0.174328404405986,
9.94496350942258));
#24364=CARTESIAN_POINT('Ctrl Pts',(-1.72141977137688,-0.176091500783687,
9.79857846054655));
#24365=CARTESIAN_POINT('Ctrl Pts',(0.902202788432801,-0.139520099979527,
9.79929936929449));
#24366=CARTESIAN_POINT('Ctrl Pts',(0.891202542074759,-0.141283196357228,
9.94355558746248));
#24367=CARTESIAN_POINT('Ctrl Pts',(0.786625228283503,-0.146572485490331,
10.3717913580854));
#24368=CARTESIAN_POINT('Ctrl Pts',(0.374692078756213,-0.153624871001134,
10.8217207397756));
#24369=CARTESIAN_POINT('Ctrl Pts',(-0.319879877211292,-0.162440352889639,
11.0603853562044));
#24370=CARTESIAN_POINT('Ctrl Pts',(-1.07349306079427,-0.171255834778144,
10.9358534528386));
#24371=CARTESIAN_POINT('Ctrl Pts',(-1.5879002756037,-0.180071316666648,
10.369048400035));
#24372=CARTESIAN_POINT('Ctrl Pts',(-1.69160147927219,-0.185360605799751,
9.9414310410581));
#24373=CARTESIAN_POINT('Ctrl Pts',(-1.70236438819101,-0.187123702177452,
9.79715692109309));
#24374=CARTESIAN_POINT('Ctrl Pts',(0.883149769673779,-0.150552301373292,
9.79784648287562));
#24375=CARTESIAN_POINT('Ctrl Pts',(0.87231047205742,-0.152315397750993,
9.9399920340605));
#24376=CARTESIAN_POINT('Ctrl Pts',(0.769263268276011,-0.157604686884096,
10.361962126063));
#24377=CARTESIAN_POINT('Ctrl Pts',(0.36335726758846,-0.164657072394899,
10.8053084217502));
#24378=CARTESIAN_POINT('Ctrl Pts',(-0.321052144861175,-0.173472554283404,
11.0404810464137));
#24379=CARTESIAN_POINT('Ctrl Pts',(-1.0636389305195,-0.182288036171909,
10.9177712161628));
#24380=CARTESIAN_POINT('Ctrl Pts',(-1.57051965989932,-0.191103518060414,
10.3592593012635));
#24381=CARTESIAN_POINT('Ctrl Pts',(-1.67270357225468,-0.196392807193516,
9.9378985726936));
#24382=CARTESIAN_POINT('Ctrl Pts',(-1.68330900500515,-0.198155903571217,
9.79573538163964));
#24383=CARTESIAN_POINT('',(0.882983735526293,-0.150579014154542,9.8));
#24384=CARTESIAN_POINT('Ctrl Pts',(0.911390797333273,-0.134200000000245,
9.80000000017706));
#24385=CARTESIAN_POINT('Ctrl Pts',(0.901922957108531,-0.139659147854633,
9.80000000017706));
#24386=CARTESIAN_POINT('Ctrl Pts',(0.892451669119078,-0.145120130049362,
9.8));
#24387=CARTESIAN_POINT('Ctrl Pts',(0.882983735526293,-0.150579014154542,
9.8));
#24388=CARTESIAN_POINT('',(-1.74047515456274,-0.165059299389922,9.8));
#24389=CARTESIAN_POINT('Ctrl Pts',(-1.74047515456274,-0.165059299389922,
9.8));
#24390=CARTESIAN_POINT('Ctrl Pts',(-1.72939729330723,-0.163296203012221,
9.94849597778708));
#24391=CARTESIAN_POINT('Ctrl Pts',(-1.69381869787564,-0.16153310663452,
10.0952061843841));
#24392=CARTESIAN_POINT('Ctrl Pts',(-1.63480228854334,-0.15977001025682,
10.2319057440229));
#24393=CARTESIAN_POINT('Ctrl Pts',(-1.51676946987873,-0.156243817501418,
10.5053048633005));
#24394=CARTESIAN_POINT('Ctrl Pts',(-1.30498539561127,-0.152717624746016,
10.7386613947454));
#24395=CARTESIAN_POINT('Ctrl Pts',(-1.04396016259108,-0.149191431990614,
10.8809748703869));
#24396=CARTESIAN_POINT('Ctrl Pts',(-0.782934929570892,-0.145665239235212,
11.0232883460284));
#24397=CARTESIAN_POINT('Ctrl Pts',(-0.472668537797981,-0.14213904647981,
11.0745587658667));
#24398=CARTESIAN_POINT('Ctrl Pts',(-0.17860719573948,-0.138612853724408,
11.0261426124902));
#24399=CARTESIAN_POINT('Ctrl Pts',(-0.0559395124477826,-0.13714190248302,
11.0059458150227));
#24400=CARTESIAN_POINT('Ctrl Pts',(0.0639082635928698,-0.135670951241633,
10.9684021475613));
#24401=CARTESIAN_POINT('Ctrl Pts',(0.176129947875697,-0.134200000000245,
10.9150835725709));
#24402=CARTESIAN_POINT('',(-1.68298373552629,-0.198103007464943,9.8));
#24403=CARTESIAN_POINT('Ctrl Pts',(-1.68298373552629,-0.198103007464943,
9.8));
#24404=CARTESIAN_POINT('Ctrl Pts',(-1.69256533649058,-0.192597003527467,
9.8));
#24405=CARTESIAN_POINT('Ctrl Pts',(-1.70215018540065,-0.187088555034124,
9.8));
#24406=CARTESIAN_POINT('Ctrl Pts',(-1.72131168622614,-0.176075287080509,
9.8));
#24407=CARTESIAN_POINT('Ctrl Pts',(-1.73089522164625,-0.170566511327364,
9.8));
#24408=CARTESIAN_POINT('Ctrl Pts',(-1.74047515456274,-0.165059299389922,
9.8));
#24409=CARTESIAN_POINT('Ctrl Pts',(0.882983744031739,-0.150579014154542,
9.80000002381835));
#24410=CARTESIAN_POINT('Ctrl Pts',(0.871962951449779,-0.152333206271826,
9.94141251268902));
#24411=CARTESIAN_POINT('Ctrl Pts',(0.768750776052023,-0.157613591144512,
10.3625218899706));
#24412=CARTESIAN_POINT('Ctrl Pts',(0.36335726758846,-0.164657072394899,
10.8053084217502));
#24413=CARTESIAN_POINT('Ctrl Pts',(-0.321052144861175,-0.173472554283404,
11.0404810464137));
#24414=CARTESIAN_POINT('Ctrl Pts',(-1.0636389305195,-0.182288036171909,
10.9177712161628));
#24415=CARTESIAN_POINT('Ctrl Pts',(-1.56950583682196,-0.191085886024989,
10.3603763929884));
#24416=CARTESIAN_POINT('Ctrl Pts',(-1.67202006066509,-0.196357543122667,
9.94070685646919));
#24417=CARTESIAN_POINT('Ctrl Pts',(-1.68298378608493,-0.198103007464943,
9.80000001577842));
#24418=CARTESIAN_POINT('Ctrl Pts',(0.361156509406693,-0.120274170443804,
8.63259693702807));
#24419=CARTESIAN_POINT('Ctrl Pts',(0.494579708156992,-0.122263574666153,
8.72773994322471));
#24420=CARTESIAN_POINT('Ctrl Pts',(0.763931929792523,-0.126905517851633,
9.00874498271484));
#24421=CARTESIAN_POINT('Ctrl Pts',(0.890509390304728,-0.131547461037113,
9.38214093563506));
#24422=CARTESIAN_POINT('Ctrl Pts',(0.907175784144597,-0.134200000000245,
9.6));
#24423=CARTESIAN_POINT('Ctrl Pts',(0.35648848307094,-0.124916113629284,
8.63914311451882));
#24424=CARTESIAN_POINT('Ctrl Pts',(0.48909342302969,-0.126905517851633,
8.73370262697521));
#24425=CARTESIAN_POINT('Ctrl Pts',(0.75679375934512,-0.131547461037113,
9.01298431665672));
#24426=CARTESIAN_POINT('Ctrl Pts',(0.882594944660462,-0.136189404222593,
9.38409030408318));
#24427=CARTESIAN_POINT('Ctrl Pts',(0.899159126715494,-0.138841943185725,
9.60061328074819));
#24428=CARTESIAN_POINT('Ctrl Pts',(0.351820456735188,-0.129558056814764,
8.64568929200957));
#24429=CARTESIAN_POINT('Ctrl Pts',(0.483607137902389,-0.131547461037113,
8.73966531072571));
#24430=CARTESIAN_POINT('Ctrl Pts',(0.749655588897719,-0.136189404222593,
9.0172236505986));
#24431=CARTESIAN_POINT('Ctrl Pts',(0.874680499016197,-0.140831347408073,
9.38603967253129));
#24432=CARTESIAN_POINT('Ctrl Pts',(0.891142469286392,-0.143483886371205,
9.60122656149638));
#24433=CARTESIAN_POINT('Ctrl Pts',(0.347152430399435,-0.134200000000245,
8.65223546950032));
#24434=CARTESIAN_POINT('Ctrl Pts',(0.478120852775088,-0.136189404222593,
8.74562799447621));
#24435=CARTESIAN_POINT('Ctrl Pts',(0.742517418450316,-0.140831347408073,
9.02146298454048));
#24436=CARTESIAN_POINT('Ctrl Pts',(0.866766053371931,-0.145473290593554,
9.3879890409794));
#24437=CARTESIAN_POINT('Ctrl Pts',(0.883125811857289,-0.148125829556685,
9.60183984224456));
#24438=CARTESIAN_POINT('',(0.882983735526293,-0.148103007464943,9.6));
#24439=CARTESIAN_POINT('Ctrl Pts',(0.882983735526293,-0.148103007464943,
9.6));
#24440=CARTESIAN_POINT('Ctrl Pts',(0.891046845655766,-0.143469594292482,
9.6));
#24441=CARTESIAN_POINT('Ctrl Pts',(0.899112255838064,-0.138834449992759,
9.6));
#24442=CARTESIAN_POINT('Ctrl Pts',(0.907175784144596,-0.134200000000245,
9.6));
#24443=CARTESIAN_POINT('Ctrl Pts',(0.347152430399435,-0.134200000000245,
8.65223546950032));
#24444=CARTESIAN_POINT('Ctrl Pts',(0.478120852775088,-0.136189404222593,
8.74562799447621));
#24445=CARTESIAN_POINT('Ctrl Pts',(0.742084116961616,-0.140823740044159,
9.02101093739862));
#24446=CARTESIAN_POINT('Ctrl Pts',(0.866358431749138,-0.145458075865725,
9.38678793547139));
#24447=CARTESIAN_POINT('Ctrl Pts',(0.882983706628455,-0.148103007464943,
9.60000000779774));
#24448=CARTESIAN_POINT('Origin',(-0.4,0.0506589891902575,9.7));
#24449=CARTESIAN_POINT('',(0.882983735526293,0.0506589891902575,9.8));
#24450=CARTESIAN_POINT('',(-1.68298373552629,-0.2,9.8));
#24451=CARTESIAN_POINT('',(-1.68298373552629,0.0506589891902575,9.8));
#24452=CARTESIAN_POINT('Origin',(-0.4,-0.2,9.7));
#24453=CARTESIAN_POINT('Origin',(-0.4,0.0506589891902575,9.7));
#24454=CARTESIAN_POINT('',(0.882983735526293,0.0506589891902575,9.6));
#24455=CARTESIAN_POINT('Origin',(-0.4,-0.3758,9.7));
#24456=CARTESIAN_POINT('',(-1.7442,-0.375799999999999,9.7));
#24457=CARTESIAN_POINT('Origin',(-0.4,-0.3758,9.7));
#24458=CARTESIAN_POINT('Origin',(-0.4,-0.3758,9.7));
#24459=CARTESIAN_POINT('Ctrl Pts',(-0.963302249831946,-0.117455697189843,
10.888459674838));
#24460=CARTESIAN_POINT('Ctrl Pts',(-1.17201968067454,-0.120250778212055,
10.7895324660635));
#24461=CARTESIAN_POINT('Ctrl Pts',(-1.5358329245996,-0.125840940256479,
10.4792728901217));
#24462=CARTESIAN_POINT('Ctrl Pts',(-1.69437043704508,-0.131431102300903,
10.0281776251649));
#24463=CARTESIAN_POINT('Ctrl Pts',(-1.71155353730395,-0.134226183323115,
9.79784243541102));
#24464=CARTESIAN_POINT('Ctrl Pts',(-0.967442787905632,-0.123037131459977,
10.8971954157908));
#24465=CARTESIAN_POINT('Ctrl Pts',(-1.17769439062363,-0.125832212482189,
10.7975410452225));
#24466=CARTESIAN_POINT('Ctrl Pts',(-1.54418183403686,-0.131422374526613,
10.4850009145922));
#24467=CARTESIAN_POINT('Ctrl Pts',(-1.70388467221392,-0.137012536571037,
10.0305898859935));
#24468=CARTESIAN_POINT('Ctrl Pts',(-1.72119407639022,-0.139807617593249,
9.79856162360734));
#24469=CARTESIAN_POINT('Ctrl Pts',(-0.971583325979318,-0.128618565730111,
10.9059311567437));
#24470=CARTESIAN_POINT('Ctrl Pts',(-1.18336910057272,-0.131413646752323,
10.8055496243816));
#24471=CARTESIAN_POINT('Ctrl Pts',(-1.55253074347412,-0.137003808796747,
10.4907289390627));
#24472=CARTESIAN_POINT('Ctrl Pts',(-1.71339890738276,-0.142593970841171,
10.033002146822));
#24473=CARTESIAN_POINT('Ctrl Pts',(-1.73083461547648,-0.145389051863383,
9.79928081180367));
#24474=CARTESIAN_POINT('Ctrl Pts',(-0.975723864053004,-0.134200000000245,
10.9146668976966));
#24475=CARTESIAN_POINT('Ctrl Pts',(-1.18904381052181,-0.136995081022457,
10.8135582035406));
#24476=CARTESIAN_POINT('Ctrl Pts',(-1.56087965291138,-0.142585243066881,
10.4964569635332));
#24477=CARTESIAN_POINT('Ctrl Pts',(-1.7229131425516,-0.148175405111305,
10.0354144076506));
#24478=CARTESIAN_POINT('Ctrl Pts',(-1.74047515456274,-0.150970486133517,
9.79999999999999));
#24479=CARTESIAN_POINT('',(-1.74047515456274,-0.150970486133517,9.8));
#24480=CARTESIAN_POINT('Ctrl Pts',(-1.74047515456274,-0.150970486133517,
9.8));
#24481=CARTESIAN_POINT('Ctrl Pts',(-1.73089506685314,-0.145446308343123,
9.8));
#24482=CARTESIAN_POINT('Ctrl Pts',(-1.72131152231243,-0.139920284562941,
9.8));
#24483=CARTESIAN_POINT('Ctrl Pts',(-1.7116177775445,-0.134330876589416,
9.8));
#24484=CARTESIAN_POINT('Ctrl Pts',(-1.71150428769636,-0.134265438426614,
9.8));
#24485=CARTESIAN_POINT('Ctrl Pts',(-1.71139079735282,-0.134200000000245,
9.8));
#24486=CARTESIAN_POINT('Ctrl Pts',(-0.975723864053004,-0.134200000000245,
10.9146668976966));
#24487=CARTESIAN_POINT('Ctrl Pts',(-1.18904381052181,-0.136995081022457,
10.8135582035406));
#24488=CARTESIAN_POINT('Ctrl Pts',(-1.3749617317166,-0.139790162044669,
10.6550075835369));
#24489=CARTESIAN_POINT('Ctrl Pts',(-1.50842906472404,-0.142585243066881,
10.4604716345644));
#24490=CARTESIAN_POINT('Ctrl Pts',(-1.64189639773149,-0.145380324089093,
10.2659356855919));
#24491=CARTESIAN_POINT('Ctrl Pts',(-1.7229131425516,-0.148175405111305,
10.0354144076506));
#24492=CARTESIAN_POINT('Ctrl Pts',(-1.74047515456274,-0.150970486133517,
9.79999999999999));
#24493=CARTESIAN_POINT('Origin',(0.6,-0.1,9.6));
#24494=CARTESIAN_POINT('',(0.906177629574171,-0.1,9.6));
#24495=CARTESIAN_POINT('Ctrl Pts',(0.906177629574171,-0.1,9.6));
#24496=CARTESIAN_POINT('Ctrl Pts',(0.923105426092673,-0.116878403916367,
9.6));
#24497=CARTESIAN_POINT('Ctrl Pts',(0.940475154562984,-0.134200000000245,
9.6));
#24498=CARTESIAN_POINT('',(0.675360404701605,-0.1,9.6));
#24499=CARTESIAN_POINT('',(0.755,-0.1,9.6));
#24500=CARTESIAN_POINT('',(0.645227248018344,-0.13,9.6));
#24501=CARTESIAN_POINT('Ctrl Pts',(0.645227248018343,-0.13,9.6));
#24502=CARTESIAN_POINT('Ctrl Pts',(0.660081620885339,-0.115213147359248,
9.6));
#24503=CARTESIAN_POINT('Ctrl Pts',(0.675360404701605,-0.1,9.6));
#24504=CARTESIAN_POINT('',(0.645227248018344,-0.2,9.6));
#24505=CARTESIAN_POINT('',(0.645227248018344,-0.265,9.6));
#24506=CARTESIAN_POINT('',(0.6,-0.2,9.6));
#24507=CARTESIAN_POINT('Origin',(-1.8,-0.1,9.6));
#24508=CARTESIAN_POINT('',(-1.44522724801834,-0.2,9.6));
#24509=CARTESIAN_POINT('',(-1.4,-0.2,9.6));
#24510=CARTESIAN_POINT('',(-1.44522724801834,-0.13,9.6));
#24511=CARTESIAN_POINT('',(-1.44522724801834,-0.265,9.6));
#24512=CARTESIAN_POINT('',(-1.4753604047016,-0.1,9.6));
#24513=CARTESIAN_POINT('Ctrl Pts',(-1.4753604047016,-0.1,9.6));
#24514=CARTESIAN_POINT('Ctrl Pts',(-1.46008162088557,-0.11521314735902,
9.6));
#24515=CARTESIAN_POINT('Ctrl Pts',(-1.44522724801834,-0.13,9.6));
#24516=CARTESIAN_POINT('',(-1.70617762957417,-0.1,9.6));
#24517=CARTESIAN_POINT('',(-0.445,-0.1,9.6));
#24518=CARTESIAN_POINT('Ctrl Pts',(-1.74047515456298,-0.134200000000245,
9.6));
#24519=CARTESIAN_POINT('Ctrl Pts',(-1.72310542608936,-0.116878403913059,
9.6));
#24520=CARTESIAN_POINT('Ctrl Pts',(-1.70617762957417,-0.1,9.6));
#24521=CARTESIAN_POINT('Origin',(-0.4,-0.255,9.7));
#24522=CARTESIAN_POINT('Origin',(-0.4,-0.3758,9.7));
#24523=CARTESIAN_POINT('Origin',(-0.4,-0.255,9.7));
#24524=CARTESIAN_POINT('',(-1.74047515456274,-0.255,9.8));
#24525=CARTESIAN_POINT('Origin',(-0.4,-0.1342,9.7));
#24526=CARTESIAN_POINT('Origin',(-1.6,-0.2,9.7));
#24527=CARTESIAN_POINT('',(-1.44522724801834,-0.2,9.8));
#24528=CARTESIAN_POINT('',(-1.8,-0.2,9.8));
#24529=CARTESIAN_POINT('',(-1.45,-0.2,9.7));
#24530=CARTESIAN_POINT('Origin',(-0.4,-0.2,9.7));
#24531=CARTESIAN_POINT('Origin',(-0.4,-0.2,9.7));
#24532=CARTESIAN_POINT('Origin',(-1.4,-0.1,9.8));
#24533=CARTESIAN_POINT('',(-1.70617762957417,-0.1,9.8));
#24534=CARTESIAN_POINT('Ctrl Pts',(-1.70617762957417,-0.1,9.8));
#24535=CARTESIAN_POINT('Ctrl Pts',(-1.72310542608936,-0.116878403913059,
9.8));
#24536=CARTESIAN_POINT('Ctrl Pts',(-1.74047515456298,-0.134200000000246,
9.8));
#24537=CARTESIAN_POINT('',(-1.4753604047016,-0.1,9.8));
#24538=CARTESIAN_POINT('',(-0.245,-0.1,9.8));
#24539=CARTESIAN_POINT('',(-1.44522724801834,-0.13,9.8));
#24540=CARTESIAN_POINT('Ctrl Pts',(-1.44522724801834,-0.13,9.8));
#24541=CARTESIAN_POINT('Ctrl Pts',(-1.46008162088557,-0.11521314735902,
9.8));
#24542=CARTESIAN_POINT('Ctrl Pts',(-1.4753604047016,-0.1,9.8));
#24543=CARTESIAN_POINT('',(-1.44522724801834,-0.265,9.8));
#24544=CARTESIAN_POINT('Origin',(0.8,-0.2,9.7));
#24545=CARTESIAN_POINT('',(0.645227248018344,-0.2,9.8));
#24546=CARTESIAN_POINT('Origin',(-0.4,-0.2,9.7));
#24547=CARTESIAN_POINT('',(1.,-0.2,9.8));
#24548=CARTESIAN_POINT('Origin',(1.,-0.1,9.8));
#24549=CARTESIAN_POINT('',(0.645227248018344,-0.13,9.8));
#24550=CARTESIAN_POINT('',(0.645227248018344,-0.265,9.8));
#24551=CARTESIAN_POINT('',(0.675360404701605,-0.1,9.8));
#24552=CARTESIAN_POINT('Ctrl Pts',(0.675360404701605,-0.1,9.8));
#24553=CARTESIAN_POINT('Ctrl Pts',(0.660081620885339,-0.115213147359248,
9.8));
#24554=CARTESIAN_POINT('Ctrl Pts',(0.645227248018343,-0.13,9.8));
#24555=CARTESIAN_POINT('',(0.906177629574171,-0.1,9.8));
#24556=CARTESIAN_POINT('',(0.955,-0.1,9.8));
#24557=CARTESIAN_POINT('Ctrl Pts',(0.940475154562984,-0.134200000000246,
9.80000000000001));
#24558=CARTESIAN_POINT('Ctrl Pts',(0.923105426092674,-0.116878403916367,
9.8));
#24559=CARTESIAN_POINT('Ctrl Pts',(0.906177629574171,-0.1,9.8));
#24560=CARTESIAN_POINT('Origin',(-0.4,-0.265,9.7));
#24561=CARTESIAN_POINT('',(-1.45,-0.4,9.7));
#24562=CARTESIAN_POINT('Origin',(-0.4,-0.4,9.7));
#24563=CARTESIAN_POINT('',(-1.45,-0.265,9.7));
#24564=CARTESIAN_POINT('Origin',(-0.4,-0.13,9.7));
#24565=CARTESIAN_POINT('Origin',(-0.4,-0.13,9.7));
#24566=CARTESIAN_POINT('Origin',(-0.4,-0.12,9.7));
#24567=CARTESIAN_POINT('Origin',(-0.4,-0.1,9.7));
#24568=CARTESIAN_POINT('Origin',(-0.4,-0.12,9.7));
#24569=CARTESIAN_POINT('Origin',(-0.4,-0.1,9.7));
#24570=CARTESIAN_POINT('Origin',(0.91,-0.1,9.7));
#24571=CARTESIAN_POINT('Origin',(-0.4,-0.1,9.7));
#24572=CARTESIAN_POINT('Origin',(0.91,-0.1,9.7));
#24573=CARTESIAN_POINT('Origin',(-0.4,-0.1,9.7));
#24574=CARTESIAN_POINT('Origin',(-0.4,-0.115,9.7));
#24575=CARTESIAN_POINT('Origin',(-0.4,-0.115,9.7));
#24576=CARTESIAN_POINT('Origin',(-0.4,-0.385,9.7));
#24577=CARTESIAN_POINT('',(-1.72,-0.4,9.7));
#24578=CARTESIAN_POINT('Origin',(-0.4,-0.4,9.7));
#24579=CARTESIAN_POINT('',(-1.735,-0.385,9.7));
#24580=CARTESIAN_POINT('Origin',(0.65,-0.4,9.7));
#38586=UNCERTAINTY_MEASURE_WITH_UNIT(LENGTH_MEASURE(0.001),#38612,
'DISTANCE_ACCURACY_VALUE',
'Maximum model space distance between geometric entities at asserted c
onnectivities');
#38595=UNCERTAINTY_MEASURE_WITH_UNIT(LENGTH_MEASURE(0.001),#38612,
'DISTANCE_ACCURACY_VALUE',
'Maximum model space distance between geometric entities at asserted c
onnectivities');
#38602=(
GEOMETRIC_REPRESENTATION_CONTEXT(3)
GLOBAL_UNCERTAINTY_ASSIGNED_CONTEXT((#38586))
GLOBAL_UNIT_ASSIGNED_CONTEXT((#38612,#38614,#38615))
REPRESENTATION_CONTEXT('','3D')
);
#38611=(
GEOMETRIC_REPRESENTATION_CONTEXT(3)
GLOBAL_UNCERTAINTY_ASSIGNED_CONTEXT((#38595))
GLOBAL_UNIT_ASSIGNED_CONTEXT((#38612,#38614,#38615))
REPRESENTATION_CONTEXT('','3D')
);
#38612=(
LENGTH_UNIT()
NAMED_UNIT(*)
SI_UNIT(.CENTI.,.METRE.)
);
#38614=(
NAMED_UNIT(*)
PLANE_ANGLE_UNIT()
SI_UNIT($,.RADIAN.)
);
#38615=(
NAMED_UNIT(*)
SI_UNIT($,.STERADIAN.)
SOLID_ANGLE_UNIT()
);
#38622=SHAPE_DEFINITION_REPRESENTATION(#38637,#38673);
#38637=PRODUCT_DEFINITION_SHAPE('',$,#38689);
#38673=SHAPE_REPRESENTATION('',(#16784),#38602);
#38682=PRODUCT_DEFINITION_CONTEXT('part definition',#38729,'design');
#38689=PRODUCT_DEFINITION('2026-10-19-02-31-35-672',
'07_Mirror_Retaining_Thread_Bezel_M27x1',#38704,#38682);
#38704=PRODUCT_DEFINITION_FORMATION('',$,#38737);
#38729=APPLICATION_CONTEXT(
'Core Data for Automotive Mechanical Design Process');
#38730=PRODUCT_CONTEXT('part definition',#38729,'mechanical');
#38737=PRODUCT('2026-10-19-02-31-35-672',
'07_Mirror_Retaining_Thread_Bezel_M27x1',$,(#38730));
#38865=COLOUR_RGB('Sky Blue',0.24,0.69,0.87);
#38866=FILL_AREA_STYLE_COLOUR('',#38865);
#38867=FILL_AREA_STYLE('',(#38866));
#38868=SURFACE_STYLE_FILL_AREA(#38867);
#38869=SURFACE_SIDE_STYLE('',(#38868));
#38870=SURFACE_STYLE_USAGE(.BOTH.,#38869);
#38871=PRESENTATION_STYLE_ASSIGNMENT((#38870));
ENDSEC;
END-ISO-10303-21;
